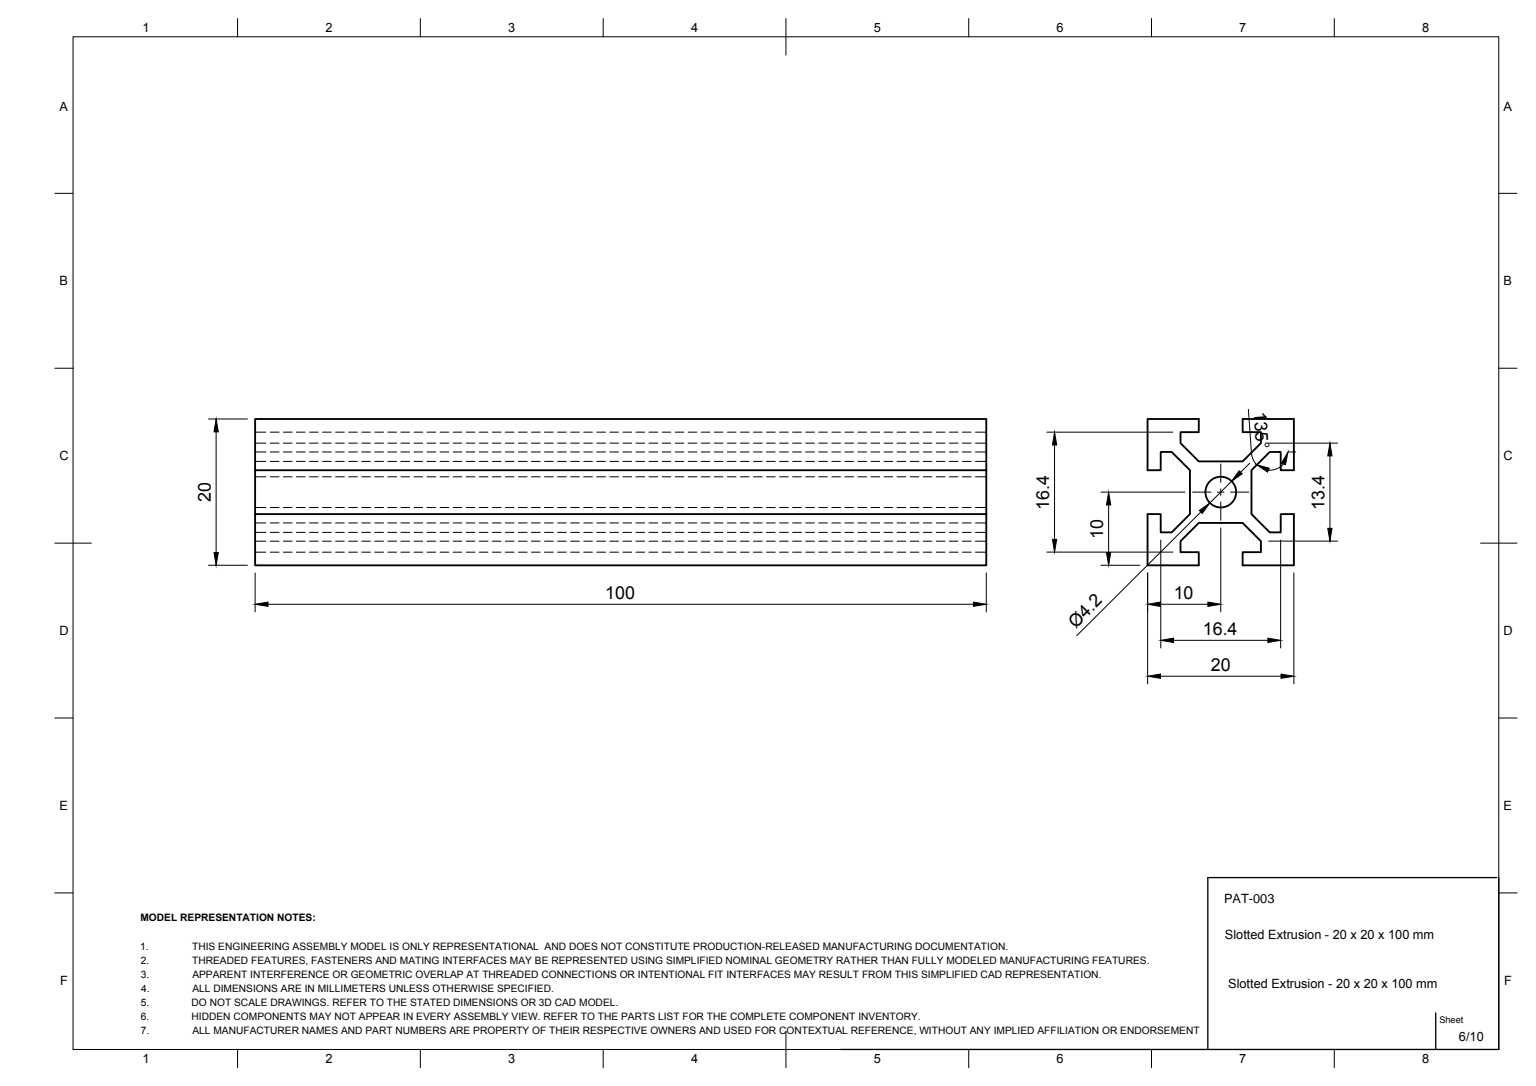
ISO-10303-21;
HEADER;
/* Generated by software containing ST-Developer
 * from STEP Tools, Inc. (www.steptools.com) 
 */

FILE_DESCRIPTION(
/* description */ ('PAT-003'),
/* implementation_level */ '2;1');

FILE_NAME(
/* name */ 'Slotted Extrusion - 20 x 20 x 100 mm.step',
/* time_stamp */ '2026-10-29T15:45:40-07:00',
/* author */ (''),
/* organization */ (''),
/* preprocessor_version */ 'ST-DEVELOPER v20.2',
/* originating_system */ 'Autodesk Translation Framework v15.17.0.0',
/* authorisation */ '');

FILE_SCHEMA (('AUTOMOTIVE_DESIGN { 1 0 10303 214 3 1 1 }'));
ENDSEC;

DATA;
#10=MECHANICAL_DESIGN_GEOMETRIC_PRESENTATION_REPRESENTATION('',(#151),#5761);
#127=SHAPE_REPRESENTATION_RELATIONSHIP('SRR','None',#5821,#139);
#139=ADVANCED_BREP_SHAPE_REPRESENTATION('',(#162),#5752);
#151=STYLED_ITEM('',(#5963),#162);
#162=MANIFOLD_SOLID_BREP('Body1',#3326);
#183=FACE_BOUND('',#640,.T.);
#184=FACE_BOUND('',#642,.T.);
#242=PLANE('',#3559);
#243=PLANE('',#3560);
#244=PLANE('',#3561);
#245=PLANE('',#3562);
#246=PLANE('',#3563);
#247=PLANE('',#3564);
#248=PLANE('',#3565);
#249=PLANE('',#3566);
#250=PLANE('',#3567);
#251=PLANE('',#3568);
#252=PLANE('',#3569);
#253=PLANE('',#3570);
#254=PLANE('',#3571);
#255=PLANE('',#3572);
#256=PLANE('',#3573);
#257=PLANE('',#3574);
#258=PLANE('',#3575);
#259=PLANE('',#3576);
#260=PLANE('',#3577);
#261=PLANE('',#3578);
#262=PLANE('',#3579);
#263=PLANE('',#3580);
#264=PLANE('',#3581);
#265=PLANE('',#3582);
#266=PLANE('',#3583);
#267=PLANE('',#3584);
#268=PLANE('',#3585);
#269=PLANE('',#3586);
#270=PLANE('',#3587);
#271=PLANE('',#3588);
#272=PLANE('',#3589);
#273=PLANE('',#3590);
#274=PLANE('',#3591);
#275=PLANE('',#3592);
#276=PLANE('',#3593);
#277=PLANE('',#3594);
#278=PLANE('',#3598);
#279=PLANE('',#3599);
#280=PLANE('',#3600);
#281=PLANE('',#3601);
#282=PLANE('',#3602);
#283=PLANE('',#3603);
#284=PLANE('',#3604);
#285=PLANE('',#3605);
#286=PLANE('',#3606);
#287=PLANE('',#3607);
#393=FACE_OUTER_BOUND('',#594,.T.);
#394=FACE_OUTER_BOUND('',#595,.T.);
#395=FACE_OUTER_BOUND('',#596,.T.);
#396=FACE_OUTER_BOUND('',#597,.T.);
#397=FACE_OUTER_BOUND('',#598,.T.);
#398=FACE_OUTER_BOUND('',#599,.T.);
#399=FACE_OUTER_BOUND('',#600,.T.);
#400=FACE_OUTER_BOUND('',#601,.T.);
#401=FACE_OUTER_BOUND('',#602,.T.);
#402=FACE_OUTER_BOUND('',#603,.T.);
#403=FACE_OUTER_BOUND('',#604,.T.);
#404=FACE_OUTER_BOUND('',#605,.T.);
#405=FACE_OUTER_BOUND('',#606,.T.);
#406=FACE_OUTER_BOUND('',#607,.T.);
#407=FACE_OUTER_BOUND('',#608,.T.);
#408=FACE_OUTER_BOUND('',#609,.T.);
#409=FACE_OUTER_BOUND('',#610,.T.);
#410=FACE_OUTER_BOUND('',#611,.T.);
#411=FACE_OUTER_BOUND('',#612,.T.);
#412=FACE_OUTER_BOUND('',#613,.T.);
#413=FACE_OUTER_BOUND('',#614,.T.);
#414=FACE_OUTER_BOUND('',#615,.T.);
#415=FACE_OUTER_BOUND('',#616,.T.);
#416=FACE_OUTER_BOUND('',#617,.T.);
#417=FACE_OUTER_BOUND('',#618,.T.);
#418=FACE_OUTER_BOUND('',#619,.T.);
#419=FACE_OUTER_BOUND('',#620,.T.);
#420=FACE_OUTER_BOUND('',#621,.T.);
#421=FACE_OUTER_BOUND('',#622,.T.);
#422=FACE_OUTER_BOUND('',#623,.T.);
#423=FACE_OUTER_BOUND('',#624,.T.);
#424=FACE_OUTER_BOUND('',#625,.T.);
#425=FACE_OUTER_BOUND('',#626,.T.);
#426=FACE_OUTER_BOUND('',#627,.T.);
#427=FACE_OUTER_BOUND('',#628,.T.);
#428=FACE_OUTER_BOUND('',#629,.T.);
#429=FACE_OUTER_BOUND('',#630,.T.);
#430=FACE_OUTER_BOUND('',#631,.T.);
#431=FACE_OUTER_BOUND('',#632,.T.);
#432=FACE_OUTER_BOUND('',#633,.T.);
#433=FACE_OUTER_BOUND('',#634,.T.);
#434=FACE_OUTER_BOUND('',#635,.T.);
#435=FACE_OUTER_BOUND('',#636,.T.);
#436=FACE_OUTER_BOUND('',#637,.T.);
#437=FACE_OUTER_BOUND('',#638,.T.);
#438=FACE_OUTER_BOUND('',#639,.T.);
#439=FACE_OUTER_BOUND('',#641,.T.);
#594=EDGE_LOOP('',(#2438,#2439,#2440,#2441));
#595=EDGE_LOOP('',(#2442,#2443,#2444,#2445));
#596=EDGE_LOOP('',(#2446,#2447,#2448,#2449));
#597=EDGE_LOOP('',(#2450,#2451,#2452,#2453));
#598=EDGE_LOOP('',(#2454,#2455,#2456,#2457));
#599=EDGE_LOOP('',(#2458,#2459,#2460,#2461));
#600=EDGE_LOOP('',(#2462,#2463,#2464,#2465));
#601=EDGE_LOOP('',(#2466,#2467,#2468,#2469));
#602=EDGE_LOOP('',(#2470,#2471,#2472,#2473));
#603=EDGE_LOOP('',(#2474,#2475,#2476,#2477));
#604=EDGE_LOOP('',(#2478,#2479,#2480,#2481));
#605=EDGE_LOOP('',(#2482,#2483,#2484,#2485));
#606=EDGE_LOOP('',(#2486,#2487,#2488,#2489));
#607=EDGE_LOOP('',(#2490,#2491,#2492,#2493));
#608=EDGE_LOOP('',(#2494,#2495,#2496,#2497));
#609=EDGE_LOOP('',(#2498,#2499,#2500,#2501));
#610=EDGE_LOOP('',(#2502,#2503,#2504,#2505));
#611=EDGE_LOOP('',(#2506,#2507,#2508,#2509));
#612=EDGE_LOOP('',(#2510,#2511,#2512,#2513));
#613=EDGE_LOOP('',(#2514,#2515,#2516,#2517));
#614=EDGE_LOOP('',(#2518,#2519,#2520,#2521));
#615=EDGE_LOOP('',(#2522,#2523,#2524,#2525));
#616=EDGE_LOOP('',(#2526,#2527,#2528,#2529));
#617=EDGE_LOOP('',(#2530,#2531,#2532,#2533));
#618=EDGE_LOOP('',(#2534,#2535,#2536,#2537));
#619=EDGE_LOOP('',(#2538,#2539,#2540,#2541));
#620=EDGE_LOOP('',(#2542,#2543,#2544,#2545));
#621=EDGE_LOOP('',(#2546,#2547,#2548,#2549));
#622=EDGE_LOOP('',(#2550,#2551,#2552,#2553));
#623=EDGE_LOOP('',(#2554,#2555,#2556,#2557));
#624=EDGE_LOOP('',(#2558,#2559,#2560,#2561));
#625=EDGE_LOOP('',(#2562,#2563,#2564,#2565));
#626=EDGE_LOOP('',(#2566,#2567,#2568,#2569));
#627=EDGE_LOOP('',(#2570,#2571,#2572,#2573));
#628=EDGE_LOOP('',(#2574,#2575,#2576,#2577));
#629=EDGE_LOOP('',(#2578,#2579,#2580,#2581));
#630=EDGE_LOOP('',(#2582,#2583,#2584,#2585));
#631=EDGE_LOOP('',(#2586,#2587,#2588,#2589));
#632=EDGE_LOOP('',(#2590,#2591,#2592,#2593));
#633=EDGE_LOOP('',(#2594,#2595,#2596,#2597));
#634=EDGE_LOOP('',(#2598,#2599,#2600,#2601));
#635=EDGE_LOOP('',(#2602,#2603,#2604,#2605));
#636=EDGE_LOOP('',(#2606,#2607,#2608,#2609));
#637=EDGE_LOOP('',(#2610,#2611,#2612,#2613));
#638=EDGE_LOOP('',(#2614,#2615,#2616,#2617));
#639=EDGE_LOOP('',(#2618,#2619,#2620,#2621,#2622,#2623,#2624,#2625,#2626,
#2627,#2628,#2629,#2630,#2631,#2632,#2633,#2634,#2635,#2636,#2637,#2638,
#2639,#2640,#2641,#2642,#2643,#2644,#2645,#2646,#2647,#2648,#2649,#2650,
#2651,#2652,#2653,#2654,#2655,#2656,#2657,#2658,#2659,#2660,#2661));
#640=EDGE_LOOP('',(#2662));
#641=EDGE_LOOP('',(#2663,#2664,#2665,#2666,#2667,#2668,#2669,#2670,#2671,
#2672,#2673,#2674,#2675,#2676,#2677,#2678,#2679,#2680,#2681,#2682,#2683,
#2684,#2685,#2686,#2687,#2688,#2689,#2690,#2691,#2692,#2693,#2694,#2695,
#2696,#2697,#2698,#2699,#2700,#2701,#2702,#2703,#2704,#2705,#2706));
#642=EDGE_LOOP('',(#2707));
#830=LINE('',#4991,#1152);
#831=LINE('',#4993,#1153);
#832=LINE('',#4995,#1154);
#833=LINE('',#4996,#1155);
#834=LINE('',#4999,#1156);
#835=LINE('',#5001,#1157);
#836=LINE('',#5002,#1158);
#837=LINE('',#5005,#1159);
#838=LINE('',#5007,#1160);
#839=LINE('',#5008,#1161);
#840=LINE('',#5011,#1162);
#841=LINE('',#5013,#1163);
#842=LINE('',#5014,#1164);
#843=LINE('',#5017,#1165);
#844=LINE('',#5019,#1166);
#845=LINE('',#5020,#1167);
#846=LINE('',#5023,#1168);
#847=LINE('',#5025,#1169);
#848=LINE('',#5026,#1170);
#849=LINE('',#5029,#1171);
#850=LINE('',#5031,#1172);
#851=LINE('',#5032,#1173);
#852=LINE('',#5035,#1174);
#853=LINE('',#5037,#1175);
#854=LINE('',#5038,#1176);
#855=LINE('',#5041,#1177);
#856=LINE('',#5043,#1178);
#857=LINE('',#5044,#1179);
#858=LINE('',#5048,#1180);
#859=LINE('',#5050,#1181);
#860=LINE('',#5052,#1182);
#861=LINE('',#5053,#1183);
#862=LINE('',#5056,#1184);
#863=LINE('',#5058,#1185);
#864=LINE('',#5059,#1186);
#865=LINE('',#5062,#1187);
#866=LINE('',#5064,#1188);
#867=LINE('',#5065,#1189);
#868=LINE('',#5068,#1190);
#869=LINE('',#5070,#1191);
#870=LINE('',#5071,#1192);
#871=LINE('',#5074,#1193);
#872=LINE('',#5076,#1194);
#873=LINE('',#5077,#1195);
#874=LINE('',#5080,#1196);
#875=LINE('',#5082,#1197);
#876=LINE('',#5083,#1198);
#877=LINE('',#5086,#1199);
#878=LINE('',#5088,#1200);
#879=LINE('',#5089,#1201);
#880=LINE('',#5092,#1202);
#881=LINE('',#5094,#1203);
#882=LINE('',#5095,#1204);
#883=LINE('',#5098,#1205);
#884=LINE('',#5100,#1206);
#885=LINE('',#5101,#1207);
#886=LINE('',#5105,#1208);
#887=LINE('',#5107,#1209);
#888=LINE('',#5109,#1210);
#889=LINE('',#5110,#1211);
#890=LINE('',#5113,#1212);
#891=LINE('',#5115,#1213);
#892=LINE('',#5116,#1214);
#893=LINE('',#5119,#1215);
#894=LINE('',#5121,#1216);
#895=LINE('',#5122,#1217);
#896=LINE('',#5125,#1218);
#897=LINE('',#5127,#1219);
#898=LINE('',#5128,#1220);
#899=LINE('',#5131,#1221);
#900=LINE('',#5133,#1222);
#901=LINE('',#5134,#1223);
#902=LINE('',#5137,#1224);
#903=LINE('',#5139,#1225);
#904=LINE('',#5140,#1226);
#905=LINE('',#5143,#1227);
#906=LINE('',#5145,#1228);
#907=LINE('',#5146,#1229);
#908=LINE('',#5149,#1230);
#909=LINE('',#5151,#1231);
#910=LINE('',#5152,#1232);
#911=LINE('',#5155,#1233);
#912=LINE('',#5157,#1234);
#913=LINE('',#5158,#1235);
#914=LINE('',#5162,#1236);
#915=LINE('',#5164,#1237);
#916=LINE('',#5166,#1238);
#917=LINE('',#5167,#1239);
#918=LINE('',#5170,#1240);
#919=LINE('',#5172,#1241);
#920=LINE('',#5173,#1242);
#921=LINE('',#5176,#1243);
#922=LINE('',#5178,#1244);
#923=LINE('',#5179,#1245);
#924=LINE('',#5182,#1246);
#925=LINE('',#5184,#1247);
#926=LINE('',#5185,#1248);
#927=LINE('',#5188,#1249);
#928=LINE('',#5190,#1250);
#929=LINE('',#5191,#1251);
#930=LINE('',#5194,#1252);
#931=LINE('',#5196,#1253);
#932=LINE('',#5197,#1254);
#933=LINE('',#5200,#1255);
#934=LINE('',#5202,#1256);
#935=LINE('',#5203,#1257);
#936=LINE('',#5206,#1258);
#937=LINE('',#5208,#1259);
#938=LINE('',#5209,#1260);
#939=LINE('',#5212,#1261);
#940=LINE('',#5214,#1262);
#941=LINE('',#5215,#1263);
#942=LINE('',#5220,#1264);
#943=LINE('',#5224,#1265);
#944=LINE('',#5226,#1266);
#945=LINE('',#5227,#1267);
#946=LINE('',#5230,#1268);
#947=LINE('',#5232,#1269);
#948=LINE('',#5233,#1270);
#949=LINE('',#5235,#1271);
#950=LINE('',#5236,#1272);
#951=LINE('',#5239,#1273);
#952=LINE('',#5241,#1274);
#953=LINE('',#5242,#1275);
#954=LINE('',#5244,#1276);
#955=LINE('',#5245,#1277);
#956=LINE('',#5248,#1278);
#957=LINE('',#5250,#1279);
#958=LINE('',#5251,#1280);
#959=LINE('',#5253,#1281);
#960=LINE('',#5254,#1282);
#961=LINE('',#5256,#1283);
#962=LINE('',#5257,#1284);
#1152=VECTOR('',#4049,1.);
#1153=VECTOR('',#4050,1.);
#1154=VECTOR('',#4051,1.);
#1155=VECTOR('',#4052,1.);
#1156=VECTOR('',#4055,1.);
#1157=VECTOR('',#4056,1.);
#1158=VECTOR('',#4057,1.);
#1159=VECTOR('',#4060,1.);
#1160=VECTOR('',#4061,1.);
#1161=VECTOR('',#4062,1.);
#1162=VECTOR('',#4065,1.);
#1163=VECTOR('',#4066,1.);
#1164=VECTOR('',#4067,1.);
#1165=VECTOR('',#4070,1.);
#1166=VECTOR('',#4071,1.);
#1167=VECTOR('',#4072,1.);
#1168=VECTOR('',#4075,1.);
#1169=VECTOR('',#4076,1.);
#1170=VECTOR('',#4077,1.);
#1171=VECTOR('',#4080,1.);
#1172=VECTOR('',#4081,1.);
#1173=VECTOR('',#4082,1.);
#1174=VECTOR('',#4085,1.);
#1175=VECTOR('',#4086,1.);
#1176=VECTOR('',#4087,1.);
#1177=VECTOR('',#4090,1.);
#1178=VECTOR('',#4091,1.);
#1179=VECTOR('',#4092,1.);
#1180=VECTOR('',#4095,1.);
#1181=VECTOR('',#4096,1.);
#1182=VECTOR('',#4097,1.);
#1183=VECTOR('',#4098,1.);
#1184=VECTOR('',#4101,1.);
#1185=VECTOR('',#4102,1.);
#1186=VECTOR('',#4103,1.);
#1187=VECTOR('',#4106,1.);
#1188=VECTOR('',#4107,1.);
#1189=VECTOR('',#4108,1.);
#1190=VECTOR('',#4111,1.);
#1191=VECTOR('',#4112,1.);
#1192=VECTOR('',#4113,1.);
#1193=VECTOR('',#4116,1.);
#1194=VECTOR('',#4117,1.);
#1195=VECTOR('',#4118,1.);
#1196=VECTOR('',#4121,1.);
#1197=VECTOR('',#4122,1.);
#1198=VECTOR('',#4123,1.);
#1199=VECTOR('',#4126,1.);
#1200=VECTOR('',#4127,1.);
#1201=VECTOR('',#4128,1.);
#1202=VECTOR('',#4131,1.);
#1203=VECTOR('',#4132,1.);
#1204=VECTOR('',#4133,1.);
#1205=VECTOR('',#4136,1.);
#1206=VECTOR('',#4137,1.);
#1207=VECTOR('',#4138,1.);
#1208=VECTOR('',#4141,1.);
#1209=VECTOR('',#4142,1.);
#1210=VECTOR('',#4143,1.);
#1211=VECTOR('',#4144,1.);
#1212=VECTOR('',#4147,1.);
#1213=VECTOR('',#4148,1.);
#1214=VECTOR('',#4149,1.);
#1215=VECTOR('',#4152,1.);
#1216=VECTOR('',#4153,1.);
#1217=VECTOR('',#4154,1.);
#1218=VECTOR('',#4157,1.);
#1219=VECTOR('',#4158,1.);
#1220=VECTOR('',#4159,1.);
#1221=VECTOR('',#4162,1.);
#1222=VECTOR('',#4163,1.);
#1223=VECTOR('',#4164,1.);
#1224=VECTOR('',#4167,1.);
#1225=VECTOR('',#4168,1.);
#1226=VECTOR('',#4169,1.);
#1227=VECTOR('',#4172,1.);
#1228=VECTOR('',#4173,1.);
#1229=VECTOR('',#4174,1.);
#1230=VECTOR('',#4177,1.);
#1231=VECTOR('',#4178,1.);
#1232=VECTOR('',#4179,1.);
#1233=VECTOR('',#4182,1.);
#1234=VECTOR('',#4183,1.);
#1235=VECTOR('',#4184,1.);
#1236=VECTOR('',#4187,1.);
#1237=VECTOR('',#4188,1.);
#1238=VECTOR('',#4189,1.);
#1239=VECTOR('',#4190,1.);
#1240=VECTOR('',#4193,1.);
#1241=VECTOR('',#4194,1.);
#1242=VECTOR('',#4195,1.);
#1243=VECTOR('',#4198,1.);
#1244=VECTOR('',#4199,1.);
#1245=VECTOR('',#4200,1.);
#1246=VECTOR('',#4203,1.);
#1247=VECTOR('',#4204,1.);
#1248=VECTOR('',#4205,1.);
#1249=VECTOR('',#4208,1.);
#1250=VECTOR('',#4209,1.);
#1251=VECTOR('',#4210,1.);
#1252=VECTOR('',#4213,1.);
#1253=VECTOR('',#4214,1.);
#1254=VECTOR('',#4215,1.);
#1255=VECTOR('',#4218,1.);
#1256=VECTOR('',#4219,1.);
#1257=VECTOR('',#4220,1.);
#1258=VECTOR('',#4223,1.);
#1259=VECTOR('',#4224,1.);
#1260=VECTOR('',#4225,1.);
#1261=VECTOR('',#4228,1.);
#1262=VECTOR('',#4229,1.);
#1263=VECTOR('',#4230,1.);
#1264=VECTOR('',#4235,0.21);
#1265=VECTOR('',#4240,1.);
#1266=VECTOR('',#4241,1.);
#1267=VECTOR('',#4242,1.);
#1268=VECTOR('',#4245,1.);
#1269=VECTOR('',#4246,1.);
#1270=VECTOR('',#4247,1.);
#1271=VECTOR('',#4250,1.);
#1272=VECTOR('',#4251,1.);
#1273=VECTOR('',#4254,1.);
#1274=VECTOR('',#4255,1.);
#1275=VECTOR('',#4256,1.);
#1276=VECTOR('',#4259,1.);
#1277=VECTOR('',#4260,1.);
#1278=VECTOR('',#4263,1.);
#1279=VECTOR('',#4264,1.);
#1280=VECTOR('',#4265,1.);
#1281=VECTOR('',#4268,1.);
#1282=VECTOR('',#4269,1.);
#1283=VECTOR('',#4272,1.);
#1284=VECTOR('',#4273,1.);
#1426=CIRCLE('',#3596,0.21);
#1427=CIRCLE('',#3597,0.21);
#1564=VERTEX_POINT('',#4989);
#1565=VERTEX_POINT('',#4990);
#1566=VERTEX_POINT('',#4992);
#1567=VERTEX_POINT('',#4994);
#1568=VERTEX_POINT('',#4998);
#1569=VERTEX_POINT('',#5000);
#1570=VERTEX_POINT('',#5004);
#1571=VERTEX_POINT('',#5006);
#1572=VERTEX_POINT('',#5010);
#1573=VERTEX_POINT('',#5012);
#1574=VERTEX_POINT('',#5016);
#1575=VERTEX_POINT('',#5018);
#1576=VERTEX_POINT('',#5022);
#1577=VERTEX_POINT('',#5024);
#1578=VERTEX_POINT('',#5028);
#1579=VERTEX_POINT('',#5030);
#1580=VERTEX_POINT('',#5034);
#1581=VERTEX_POINT('',#5036);
#1582=VERTEX_POINT('',#5040);
#1583=VERTEX_POINT('',#5042);
#1584=VERTEX_POINT('',#5046);
#1585=VERTEX_POINT('',#5047);
#1586=VERTEX_POINT('',#5049);
#1587=VERTEX_POINT('',#5051);
#1588=VERTEX_POINT('',#5055);
#1589=VERTEX_POINT('',#5057);
#1590=VERTEX_POINT('',#5061);
#1591=VERTEX_POINT('',#5063);
#1592=VERTEX_POINT('',#5067);
#1593=VERTEX_POINT('',#5069);
#1594=VERTEX_POINT('',#5073);
#1595=VERTEX_POINT('',#5075);
#1596=VERTEX_POINT('',#5079);
#1597=VERTEX_POINT('',#5081);
#1598=VERTEX_POINT('',#5085);
#1599=VERTEX_POINT('',#5087);
#1600=VERTEX_POINT('',#5091);
#1601=VERTEX_POINT('',#5093);
#1602=VERTEX_POINT('',#5097);
#1603=VERTEX_POINT('',#5099);
#1604=VERTEX_POINT('',#5103);
#1605=VERTEX_POINT('',#5104);
#1606=VERTEX_POINT('',#5106);
#1607=VERTEX_POINT('',#5108);
#1608=VERTEX_POINT('',#5112);
#1609=VERTEX_POINT('',#5114);
#1610=VERTEX_POINT('',#5118);
#1611=VERTEX_POINT('',#5120);
#1612=VERTEX_POINT('',#5124);
#1613=VERTEX_POINT('',#5126);
#1614=VERTEX_POINT('',#5130);
#1615=VERTEX_POINT('',#5132);
#1616=VERTEX_POINT('',#5136);
#1617=VERTEX_POINT('',#5138);
#1618=VERTEX_POINT('',#5142);
#1619=VERTEX_POINT('',#5144);
#1620=VERTEX_POINT('',#5148);
#1621=VERTEX_POINT('',#5150);
#1622=VERTEX_POINT('',#5154);
#1623=VERTEX_POINT('',#5156);
#1624=VERTEX_POINT('',#5160);
#1625=VERTEX_POINT('',#5161);
#1626=VERTEX_POINT('',#5163);
#1627=VERTEX_POINT('',#5165);
#1628=VERTEX_POINT('',#5169);
#1629=VERTEX_POINT('',#5171);
#1630=VERTEX_POINT('',#5175);
#1631=VERTEX_POINT('',#5177);
#1632=VERTEX_POINT('',#5181);
#1633=VERTEX_POINT('',#5183);
#1634=VERTEX_POINT('',#5187);
#1635=VERTEX_POINT('',#5189);
#1636=VERTEX_POINT('',#5193);
#1637=VERTEX_POINT('',#5195);
#1638=VERTEX_POINT('',#5199);
#1639=VERTEX_POINT('',#5201);
#1640=VERTEX_POINT('',#5205);
#1641=VERTEX_POINT('',#5207);
#1642=VERTEX_POINT('',#5211);
#1643=VERTEX_POINT('',#5213);
#1644=VERTEX_POINT('',#5217);
#1645=VERTEX_POINT('',#5219);
#1646=VERTEX_POINT('',#5223);
#1647=VERTEX_POINT('',#5225);
#1648=VERTEX_POINT('',#5229);
#1649=VERTEX_POINT('',#5231);
#1650=VERTEX_POINT('',#5238);
#1651=VERTEX_POINT('',#5240);
#1652=VERTEX_POINT('',#5247);
#1653=VERTEX_POINT('',#5249);
#1890=EDGE_CURVE('',#1564,#1565,#830,.T.);
#1891=EDGE_CURVE('',#1564,#1566,#831,.T.);
#1892=EDGE_CURVE('',#1567,#1566,#832,.T.);
#1893=EDGE_CURVE('',#1565,#1567,#833,.T.);
#1894=EDGE_CURVE('',#1568,#1564,#834,.T.);
#1895=EDGE_CURVE('',#1568,#1569,#835,.T.);
#1896=EDGE_CURVE('',#1566,#1569,#836,.T.);
#1897=EDGE_CURVE('',#1570,#1568,#837,.T.);
#1898=EDGE_CURVE('',#1570,#1571,#838,.T.);
#1899=EDGE_CURVE('',#1569,#1571,#839,.T.);
#1900=EDGE_CURVE('',#1572,#1570,#840,.T.);
#1901=EDGE_CURVE('',#1572,#1573,#841,.T.);
#1902=EDGE_CURVE('',#1571,#1573,#842,.T.);
#1903=EDGE_CURVE('',#1574,#1572,#843,.T.);
#1904=EDGE_CURVE('',#1574,#1575,#844,.T.);
#1905=EDGE_CURVE('',#1573,#1575,#845,.T.);
#1906=EDGE_CURVE('',#1576,#1574,#846,.T.);
#1907=EDGE_CURVE('',#1576,#1577,#847,.T.);
#1908=EDGE_CURVE('',#1575,#1577,#848,.T.);
#1909=EDGE_CURVE('',#1578,#1576,#849,.T.);
#1910=EDGE_CURVE('',#1578,#1579,#850,.T.);
#1911=EDGE_CURVE('',#1577,#1579,#851,.T.);
#1912=EDGE_CURVE('',#1580,#1578,#852,.T.);
#1913=EDGE_CURVE('',#1580,#1581,#853,.T.);
#1914=EDGE_CURVE('',#1579,#1581,#854,.T.);
#1915=EDGE_CURVE('',#1582,#1580,#855,.T.);
#1916=EDGE_CURVE('',#1583,#1582,#856,.T.);
#1917=EDGE_CURVE('',#1581,#1583,#857,.T.);
#1918=EDGE_CURVE('',#1584,#1585,#858,.T.);
#1919=EDGE_CURVE('',#1584,#1586,#859,.T.);
#1920=EDGE_CURVE('',#1587,#1586,#860,.T.);
#1921=EDGE_CURVE('',#1585,#1587,#861,.T.);
#1922=EDGE_CURVE('',#1588,#1584,#862,.T.);
#1923=EDGE_CURVE('',#1588,#1589,#863,.T.);
#1924=EDGE_CURVE('',#1586,#1589,#864,.T.);
#1925=EDGE_CURVE('',#1590,#1588,#865,.T.);
#1926=EDGE_CURVE('',#1590,#1591,#866,.T.);
#1927=EDGE_CURVE('',#1589,#1591,#867,.T.);
#1928=EDGE_CURVE('',#1592,#1590,#868,.T.);
#1929=EDGE_CURVE('',#1592,#1593,#869,.T.);
#1930=EDGE_CURVE('',#1591,#1593,#870,.T.);
#1931=EDGE_CURVE('',#1594,#1592,#871,.T.);
#1932=EDGE_CURVE('',#1594,#1595,#872,.T.);
#1933=EDGE_CURVE('',#1593,#1595,#873,.T.);
#1934=EDGE_CURVE('',#1596,#1594,#874,.T.);
#1935=EDGE_CURVE('',#1596,#1597,#875,.T.);
#1936=EDGE_CURVE('',#1595,#1597,#876,.T.);
#1937=EDGE_CURVE('',#1598,#1596,#877,.T.);
#1938=EDGE_CURVE('',#1598,#1599,#878,.T.);
#1939=EDGE_CURVE('',#1597,#1599,#879,.T.);
#1940=EDGE_CURVE('',#1600,#1598,#880,.T.);
#1941=EDGE_CURVE('',#1600,#1601,#881,.T.);
#1942=EDGE_CURVE('',#1599,#1601,#882,.T.);
#1943=EDGE_CURVE('',#1602,#1600,#883,.T.);
#1944=EDGE_CURVE('',#1603,#1602,#884,.T.);
#1945=EDGE_CURVE('',#1601,#1603,#885,.T.);
#1946=EDGE_CURVE('',#1604,#1605,#886,.T.);
#1947=EDGE_CURVE('',#1604,#1606,#887,.T.);
#1948=EDGE_CURVE('',#1607,#1606,#888,.T.);
#1949=EDGE_CURVE('',#1605,#1607,#889,.T.);
#1950=EDGE_CURVE('',#1608,#1604,#890,.T.);
#1951=EDGE_CURVE('',#1608,#1609,#891,.T.);
#1952=EDGE_CURVE('',#1606,#1609,#892,.T.);
#1953=EDGE_CURVE('',#1610,#1608,#893,.T.);
#1954=EDGE_CURVE('',#1610,#1611,#894,.T.);
#1955=EDGE_CURVE('',#1609,#1611,#895,.T.);
#1956=EDGE_CURVE('',#1612,#1610,#896,.T.);
#1957=EDGE_CURVE('',#1612,#1613,#897,.T.);
#1958=EDGE_CURVE('',#1611,#1613,#898,.T.);
#1959=EDGE_CURVE('',#1614,#1612,#899,.T.);
#1960=EDGE_CURVE('',#1614,#1615,#900,.T.);
#1961=EDGE_CURVE('',#1613,#1615,#901,.T.);
#1962=EDGE_CURVE('',#1616,#1614,#902,.T.);
#1963=EDGE_CURVE('',#1616,#1617,#903,.T.);
#1964=EDGE_CURVE('',#1615,#1617,#904,.T.);
#1965=EDGE_CURVE('',#1618,#1616,#905,.T.);
#1966=EDGE_CURVE('',#1618,#1619,#906,.T.);
#1967=EDGE_CURVE('',#1617,#1619,#907,.T.);
#1968=EDGE_CURVE('',#1620,#1618,#908,.T.);
#1969=EDGE_CURVE('',#1620,#1621,#909,.T.);
#1970=EDGE_CURVE('',#1619,#1621,#910,.T.);
#1971=EDGE_CURVE('',#1622,#1620,#911,.T.);
#1972=EDGE_CURVE('',#1623,#1622,#912,.T.);
#1973=EDGE_CURVE('',#1621,#1623,#913,.T.);
#1974=EDGE_CURVE('',#1624,#1625,#914,.T.);
#1975=EDGE_CURVE('',#1624,#1626,#915,.T.);
#1976=EDGE_CURVE('',#1627,#1626,#916,.T.);
#1977=EDGE_CURVE('',#1625,#1627,#917,.T.);
#1978=EDGE_CURVE('',#1628,#1624,#918,.T.);
#1979=EDGE_CURVE('',#1628,#1629,#919,.T.);
#1980=EDGE_CURVE('',#1626,#1629,#920,.T.);
#1981=EDGE_CURVE('',#1630,#1628,#921,.T.);
#1982=EDGE_CURVE('',#1630,#1631,#922,.T.);
#1983=EDGE_CURVE('',#1629,#1631,#923,.T.);
#1984=EDGE_CURVE('',#1632,#1630,#924,.T.);
#1985=EDGE_CURVE('',#1632,#1633,#925,.T.);
#1986=EDGE_CURVE('',#1631,#1633,#926,.T.);
#1987=EDGE_CURVE('',#1634,#1632,#927,.T.);
#1988=EDGE_CURVE('',#1634,#1635,#928,.T.);
#1989=EDGE_CURVE('',#1633,#1635,#929,.T.);
#1990=EDGE_CURVE('',#1636,#1634,#930,.T.);
#1991=EDGE_CURVE('',#1636,#1637,#931,.T.);
#1992=EDGE_CURVE('',#1635,#1637,#932,.T.);
#1993=EDGE_CURVE('',#1638,#1636,#933,.T.);
#1994=EDGE_CURVE('',#1638,#1639,#934,.T.);
#1995=EDGE_CURVE('',#1637,#1639,#935,.T.);
#1996=EDGE_CURVE('',#1640,#1638,#936,.T.);
#1997=EDGE_CURVE('',#1640,#1641,#937,.T.);
#1998=EDGE_CURVE('',#1639,#1641,#938,.T.);
#1999=EDGE_CURVE('',#1642,#1640,#939,.T.);
#2000=EDGE_CURVE('',#1643,#1642,#940,.T.);
#2001=EDGE_CURVE('',#1641,#1643,#941,.T.);
#2002=EDGE_CURVE('',#1644,#1644,#1426,.T.);
#2003=EDGE_CURVE('',#1644,#1645,#942,.T.);
#2004=EDGE_CURVE('',#1645,#1645,#1427,.T.);
#2005=EDGE_CURVE('',#1582,#1646,#943,.T.);
#2006=EDGE_CURVE('',#1646,#1647,#944,.T.);
#2007=EDGE_CURVE('',#1583,#1647,#945,.T.);
#2008=EDGE_CURVE('',#1648,#1567,#946,.T.);
#2009=EDGE_CURVE('',#1649,#1648,#947,.T.);
#2010=EDGE_CURVE('',#1649,#1565,#948,.T.);
#2011=EDGE_CURVE('',#1602,#1649,#949,.T.);
#2012=EDGE_CURVE('',#1603,#1648,#950,.T.);
#2013=EDGE_CURVE('',#1650,#1587,#951,.T.);
#2014=EDGE_CURVE('',#1651,#1650,#952,.T.);
#2015=EDGE_CURVE('',#1651,#1585,#953,.T.);
#2016=EDGE_CURVE('',#1622,#1651,#954,.T.);
#2017=EDGE_CURVE('',#1623,#1650,#955,.T.);
#2018=EDGE_CURVE('',#1652,#1607,#956,.T.);
#2019=EDGE_CURVE('',#1653,#1652,#957,.T.);
#2020=EDGE_CURVE('',#1653,#1605,#958,.T.);
#2021=EDGE_CURVE('',#1642,#1653,#959,.T.);
#2022=EDGE_CURVE('',#1643,#1652,#960,.T.);
#2023=EDGE_CURVE('',#1647,#1627,#961,.T.);
#2024=EDGE_CURVE('',#1646,#1625,#962,.T.);
#2438=ORIENTED_EDGE('',*,*,#1890,.F.);
#2439=ORIENTED_EDGE('',*,*,#1891,.T.);
#2440=ORIENTED_EDGE('',*,*,#1892,.F.);
#2441=ORIENTED_EDGE('',*,*,#1893,.F.);
#2442=ORIENTED_EDGE('',*,*,#1894,.F.);
#2443=ORIENTED_EDGE('',*,*,#1895,.T.);
#2444=ORIENTED_EDGE('',*,*,#1896,.F.);
#2445=ORIENTED_EDGE('',*,*,#1891,.F.);
#2446=ORIENTED_EDGE('',*,*,#1897,.F.);
#2447=ORIENTED_EDGE('',*,*,#1898,.T.);
#2448=ORIENTED_EDGE('',*,*,#1899,.F.);
#2449=ORIENTED_EDGE('',*,*,#1895,.F.);
#2450=ORIENTED_EDGE('',*,*,#1900,.F.);
#2451=ORIENTED_EDGE('',*,*,#1901,.T.);
#2452=ORIENTED_EDGE('',*,*,#1902,.F.);
#2453=ORIENTED_EDGE('',*,*,#1898,.F.);
#2454=ORIENTED_EDGE('',*,*,#1903,.F.);
#2455=ORIENTED_EDGE('',*,*,#1904,.T.);
#2456=ORIENTED_EDGE('',*,*,#1905,.F.);
#2457=ORIENTED_EDGE('',*,*,#1901,.F.);
#2458=ORIENTED_EDGE('',*,*,#1906,.F.);
#2459=ORIENTED_EDGE('',*,*,#1907,.T.);
#2460=ORIENTED_EDGE('',*,*,#1908,.F.);
#2461=ORIENTED_EDGE('',*,*,#1904,.F.);
#2462=ORIENTED_EDGE('',*,*,#1909,.F.);
#2463=ORIENTED_EDGE('',*,*,#1910,.T.);
#2464=ORIENTED_EDGE('',*,*,#1911,.F.);
#2465=ORIENTED_EDGE('',*,*,#1907,.F.);
#2466=ORIENTED_EDGE('',*,*,#1912,.F.);
#2467=ORIENTED_EDGE('',*,*,#1913,.T.);
#2468=ORIENTED_EDGE('',*,*,#1914,.F.);
#2469=ORIENTED_EDGE('',*,*,#1910,.F.);
#2470=ORIENTED_EDGE('',*,*,#1915,.F.);
#2471=ORIENTED_EDGE('',*,*,#1916,.F.);
#2472=ORIENTED_EDGE('',*,*,#1917,.F.);
#2473=ORIENTED_EDGE('',*,*,#1913,.F.);
#2474=ORIENTED_EDGE('',*,*,#1918,.F.);
#2475=ORIENTED_EDGE('',*,*,#1919,.T.);
#2476=ORIENTED_EDGE('',*,*,#1920,.F.);
#2477=ORIENTED_EDGE('',*,*,#1921,.F.);
#2478=ORIENTED_EDGE('',*,*,#1922,.F.);
#2479=ORIENTED_EDGE('',*,*,#1923,.T.);
#2480=ORIENTED_EDGE('',*,*,#1924,.F.);
#2481=ORIENTED_EDGE('',*,*,#1919,.F.);
#2482=ORIENTED_EDGE('',*,*,#1925,.F.);
#2483=ORIENTED_EDGE('',*,*,#1926,.T.);
#2484=ORIENTED_EDGE('',*,*,#1927,.F.);
#2485=ORIENTED_EDGE('',*,*,#1923,.F.);
#2486=ORIENTED_EDGE('',*,*,#1928,.F.);
#2487=ORIENTED_EDGE('',*,*,#1929,.T.);
#2488=ORIENTED_EDGE('',*,*,#1930,.F.);
#2489=ORIENTED_EDGE('',*,*,#1926,.F.);
#2490=ORIENTED_EDGE('',*,*,#1931,.F.);
#2491=ORIENTED_EDGE('',*,*,#1932,.T.);
#2492=ORIENTED_EDGE('',*,*,#1933,.F.);
#2493=ORIENTED_EDGE('',*,*,#1929,.F.);
#2494=ORIENTED_EDGE('',*,*,#1934,.F.);
#2495=ORIENTED_EDGE('',*,*,#1935,.T.);
#2496=ORIENTED_EDGE('',*,*,#1936,.F.);
#2497=ORIENTED_EDGE('',*,*,#1932,.F.);
#2498=ORIENTED_EDGE('',*,*,#1937,.F.);
#2499=ORIENTED_EDGE('',*,*,#1938,.T.);
#2500=ORIENTED_EDGE('',*,*,#1939,.F.);
#2501=ORIENTED_EDGE('',*,*,#1935,.F.);
#2502=ORIENTED_EDGE('',*,*,#1940,.F.);
#2503=ORIENTED_EDGE('',*,*,#1941,.T.);
#2504=ORIENTED_EDGE('',*,*,#1942,.F.);
#2505=ORIENTED_EDGE('',*,*,#1938,.F.);
#2506=ORIENTED_EDGE('',*,*,#1943,.F.);
#2507=ORIENTED_EDGE('',*,*,#1944,.F.);
#2508=ORIENTED_EDGE('',*,*,#1945,.F.);
#2509=ORIENTED_EDGE('',*,*,#1941,.F.);
#2510=ORIENTED_EDGE('',*,*,#1946,.F.);
#2511=ORIENTED_EDGE('',*,*,#1947,.T.);
#2512=ORIENTED_EDGE('',*,*,#1948,.F.);
#2513=ORIENTED_EDGE('',*,*,#1949,.F.);
#2514=ORIENTED_EDGE('',*,*,#1950,.F.);
#2515=ORIENTED_EDGE('',*,*,#1951,.T.);
#2516=ORIENTED_EDGE('',*,*,#1952,.F.);
#2517=ORIENTED_EDGE('',*,*,#1947,.F.);
#2518=ORIENTED_EDGE('',*,*,#1953,.F.);
#2519=ORIENTED_EDGE('',*,*,#1954,.T.);
#2520=ORIENTED_EDGE('',*,*,#1955,.F.);
#2521=ORIENTED_EDGE('',*,*,#1951,.F.);
#2522=ORIENTED_EDGE('',*,*,#1956,.F.);
#2523=ORIENTED_EDGE('',*,*,#1957,.T.);
#2524=ORIENTED_EDGE('',*,*,#1958,.F.);
#2525=ORIENTED_EDGE('',*,*,#1954,.F.);
#2526=ORIENTED_EDGE('',*,*,#1959,.F.);
#2527=ORIENTED_EDGE('',*,*,#1960,.T.);
#2528=ORIENTED_EDGE('',*,*,#1961,.F.);
#2529=ORIENTED_EDGE('',*,*,#1957,.F.);
#2530=ORIENTED_EDGE('',*,*,#1962,.F.);
#2531=ORIENTED_EDGE('',*,*,#1963,.T.);
#2532=ORIENTED_EDGE('',*,*,#1964,.F.);
#2533=ORIENTED_EDGE('',*,*,#1960,.F.);
#2534=ORIENTED_EDGE('',*,*,#1965,.F.);
#2535=ORIENTED_EDGE('',*,*,#1966,.T.);
#2536=ORIENTED_EDGE('',*,*,#1967,.F.);
#2537=ORIENTED_EDGE('',*,*,#1963,.F.);
#2538=ORIENTED_EDGE('',*,*,#1968,.F.);
#2539=ORIENTED_EDGE('',*,*,#1969,.T.);
#2540=ORIENTED_EDGE('',*,*,#1970,.F.);
#2541=ORIENTED_EDGE('',*,*,#1966,.F.);
#2542=ORIENTED_EDGE('',*,*,#1971,.F.);
#2543=ORIENTED_EDGE('',*,*,#1972,.F.);
#2544=ORIENTED_EDGE('',*,*,#1973,.F.);
#2545=ORIENTED_EDGE('',*,*,#1969,.F.);
#2546=ORIENTED_EDGE('',*,*,#1974,.F.);
#2547=ORIENTED_EDGE('',*,*,#1975,.T.);
#2548=ORIENTED_EDGE('',*,*,#1976,.F.);
#2549=ORIENTED_EDGE('',*,*,#1977,.F.);
#2550=ORIENTED_EDGE('',*,*,#1978,.F.);
#2551=ORIENTED_EDGE('',*,*,#1979,.T.);
#2552=ORIENTED_EDGE('',*,*,#1980,.F.);
#2553=ORIENTED_EDGE('',*,*,#1975,.F.);
#2554=ORIENTED_EDGE('',*,*,#1981,.F.);
#2555=ORIENTED_EDGE('',*,*,#1982,.T.);
#2556=ORIENTED_EDGE('',*,*,#1983,.F.);
#2557=ORIENTED_EDGE('',*,*,#1979,.F.);
#2558=ORIENTED_EDGE('',*,*,#1984,.F.);
#2559=ORIENTED_EDGE('',*,*,#1985,.T.);
#2560=ORIENTED_EDGE('',*,*,#1986,.F.);
#2561=ORIENTED_EDGE('',*,*,#1982,.F.);
#2562=ORIENTED_EDGE('',*,*,#1987,.F.);
#2563=ORIENTED_EDGE('',*,*,#1988,.T.);
#2564=ORIENTED_EDGE('',*,*,#1989,.F.);
#2565=ORIENTED_EDGE('',*,*,#1985,.F.);
#2566=ORIENTED_EDGE('',*,*,#1990,.F.);
#2567=ORIENTED_EDGE('',*,*,#1991,.T.);
#2568=ORIENTED_EDGE('',*,*,#1992,.F.);
#2569=ORIENTED_EDGE('',*,*,#1988,.F.);
#2570=ORIENTED_EDGE('',*,*,#1993,.F.);
#2571=ORIENTED_EDGE('',*,*,#1994,.T.);
#2572=ORIENTED_EDGE('',*,*,#1995,.F.);
#2573=ORIENTED_EDGE('',*,*,#1991,.F.);
#2574=ORIENTED_EDGE('',*,*,#1996,.F.);
#2575=ORIENTED_EDGE('',*,*,#1997,.T.);
#2576=ORIENTED_EDGE('',*,*,#1998,.F.);
#2577=ORIENTED_EDGE('',*,*,#1994,.F.);
#2578=ORIENTED_EDGE('',*,*,#1999,.F.);
#2579=ORIENTED_EDGE('',*,*,#2000,.F.);
#2580=ORIENTED_EDGE('',*,*,#2001,.F.);
#2581=ORIENTED_EDGE('',*,*,#1997,.F.);
#2582=ORIENTED_EDGE('',*,*,#2002,.F.);
#2583=ORIENTED_EDGE('',*,*,#2003,.T.);
#2584=ORIENTED_EDGE('',*,*,#2004,.F.);
#2585=ORIENTED_EDGE('',*,*,#2003,.F.);
#2586=ORIENTED_EDGE('',*,*,#1916,.T.);
#2587=ORIENTED_EDGE('',*,*,#2005,.T.);
#2588=ORIENTED_EDGE('',*,*,#2006,.T.);
#2589=ORIENTED_EDGE('',*,*,#2007,.F.);
#2590=ORIENTED_EDGE('',*,*,#1893,.T.);
#2591=ORIENTED_EDGE('',*,*,#2008,.F.);
#2592=ORIENTED_EDGE('',*,*,#2009,.F.);
#2593=ORIENTED_EDGE('',*,*,#2010,.T.);
#2594=ORIENTED_EDGE('',*,*,#1944,.T.);
#2595=ORIENTED_EDGE('',*,*,#2011,.T.);
#2596=ORIENTED_EDGE('',*,*,#2009,.T.);
#2597=ORIENTED_EDGE('',*,*,#2012,.F.);
#2598=ORIENTED_EDGE('',*,*,#1921,.T.);
#2599=ORIENTED_EDGE('',*,*,#2013,.F.);
#2600=ORIENTED_EDGE('',*,*,#2014,.F.);
#2601=ORIENTED_EDGE('',*,*,#2015,.T.);
#2602=ORIENTED_EDGE('',*,*,#1972,.T.);
#2603=ORIENTED_EDGE('',*,*,#2016,.T.);
#2604=ORIENTED_EDGE('',*,*,#2014,.T.);
#2605=ORIENTED_EDGE('',*,*,#2017,.F.);
#2606=ORIENTED_EDGE('',*,*,#1949,.T.);
#2607=ORIENTED_EDGE('',*,*,#2018,.F.);
#2608=ORIENTED_EDGE('',*,*,#2019,.F.);
#2609=ORIENTED_EDGE('',*,*,#2020,.T.);
#2610=ORIENTED_EDGE('',*,*,#2000,.T.);
#2611=ORIENTED_EDGE('',*,*,#2021,.T.);
#2612=ORIENTED_EDGE('',*,*,#2019,.T.);
#2613=ORIENTED_EDGE('',*,*,#2022,.F.);
#2614=ORIENTED_EDGE('',*,*,#1977,.T.);
#2615=ORIENTED_EDGE('',*,*,#2023,.F.);
#2616=ORIENTED_EDGE('',*,*,#2006,.F.);
#2617=ORIENTED_EDGE('',*,*,#2024,.T.);
#2618=ORIENTED_EDGE('',*,*,#1892,.T.);
#2619=ORIENTED_EDGE('',*,*,#1896,.T.);
#2620=ORIENTED_EDGE('',*,*,#1899,.T.);
#2621=ORIENTED_EDGE('',*,*,#1902,.T.);
#2622=ORIENTED_EDGE('',*,*,#1905,.T.);
#2623=ORIENTED_EDGE('',*,*,#1908,.T.);
#2624=ORIENTED_EDGE('',*,*,#1911,.T.);
#2625=ORIENTED_EDGE('',*,*,#1914,.T.);
#2626=ORIENTED_EDGE('',*,*,#1917,.T.);
#2627=ORIENTED_EDGE('',*,*,#2007,.T.);
#2628=ORIENTED_EDGE('',*,*,#2023,.T.);
#2629=ORIENTED_EDGE('',*,*,#1976,.T.);
#2630=ORIENTED_EDGE('',*,*,#1980,.T.);
#2631=ORIENTED_EDGE('',*,*,#1983,.T.);
#2632=ORIENTED_EDGE('',*,*,#1986,.T.);
#2633=ORIENTED_EDGE('',*,*,#1989,.T.);
#2634=ORIENTED_EDGE('',*,*,#1992,.T.);
#2635=ORIENTED_EDGE('',*,*,#1995,.T.);
#2636=ORIENTED_EDGE('',*,*,#1998,.T.);
#2637=ORIENTED_EDGE('',*,*,#2001,.T.);
#2638=ORIENTED_EDGE('',*,*,#2022,.T.);
#2639=ORIENTED_EDGE('',*,*,#2018,.T.);
#2640=ORIENTED_EDGE('',*,*,#1948,.T.);
#2641=ORIENTED_EDGE('',*,*,#1952,.T.);
#2642=ORIENTED_EDGE('',*,*,#1955,.T.);
#2643=ORIENTED_EDGE('',*,*,#1958,.T.);
#2644=ORIENTED_EDGE('',*,*,#1961,.T.);
#2645=ORIENTED_EDGE('',*,*,#1964,.T.);
#2646=ORIENTED_EDGE('',*,*,#1967,.T.);
#2647=ORIENTED_EDGE('',*,*,#1970,.T.);
#2648=ORIENTED_EDGE('',*,*,#1973,.T.);
#2649=ORIENTED_EDGE('',*,*,#2017,.T.);
#2650=ORIENTED_EDGE('',*,*,#2013,.T.);
#2651=ORIENTED_EDGE('',*,*,#1920,.T.);
#2652=ORIENTED_EDGE('',*,*,#1924,.T.);
#2653=ORIENTED_EDGE('',*,*,#1927,.T.);
#2654=ORIENTED_EDGE('',*,*,#1930,.T.);
#2655=ORIENTED_EDGE('',*,*,#1933,.T.);
#2656=ORIENTED_EDGE('',*,*,#1936,.T.);
#2657=ORIENTED_EDGE('',*,*,#1939,.T.);
#2658=ORIENTED_EDGE('',*,*,#1942,.T.);
#2659=ORIENTED_EDGE('',*,*,#1945,.T.);
#2660=ORIENTED_EDGE('',*,*,#2012,.T.);
#2661=ORIENTED_EDGE('',*,*,#2008,.T.);
#2662=ORIENTED_EDGE('',*,*,#2004,.T.);
#2663=ORIENTED_EDGE('',*,*,#1890,.T.);
#2664=ORIENTED_EDGE('',*,*,#2010,.F.);
#2665=ORIENTED_EDGE('',*,*,#2011,.F.);
#2666=ORIENTED_EDGE('',*,*,#1943,.T.);
#2667=ORIENTED_EDGE('',*,*,#1940,.T.);
#2668=ORIENTED_EDGE('',*,*,#1937,.T.);
#2669=ORIENTED_EDGE('',*,*,#1934,.T.);
#2670=ORIENTED_EDGE('',*,*,#1931,.T.);
#2671=ORIENTED_EDGE('',*,*,#1928,.T.);
#2672=ORIENTED_EDGE('',*,*,#1925,.T.);
#2673=ORIENTED_EDGE('',*,*,#1922,.T.);
#2674=ORIENTED_EDGE('',*,*,#1918,.T.);
#2675=ORIENTED_EDGE('',*,*,#2015,.F.);
#2676=ORIENTED_EDGE('',*,*,#2016,.F.);
#2677=ORIENTED_EDGE('',*,*,#1971,.T.);
#2678=ORIENTED_EDGE('',*,*,#1968,.T.);
#2679=ORIENTED_EDGE('',*,*,#1965,.T.);
#2680=ORIENTED_EDGE('',*,*,#1962,.T.);
#2681=ORIENTED_EDGE('',*,*,#1959,.T.);
#2682=ORIENTED_EDGE('',*,*,#1956,.T.);
#2683=ORIENTED_EDGE('',*,*,#1953,.T.);
#2684=ORIENTED_EDGE('',*,*,#1950,.T.);
#2685=ORIENTED_EDGE('',*,*,#1946,.T.);
#2686=ORIENTED_EDGE('',*,*,#2020,.F.);
#2687=ORIENTED_EDGE('',*,*,#2021,.F.);
#2688=ORIENTED_EDGE('',*,*,#1999,.T.);
#2689=ORIENTED_EDGE('',*,*,#1996,.T.);
#2690=ORIENTED_EDGE('',*,*,#1993,.T.);
#2691=ORIENTED_EDGE('',*,*,#1990,.T.);
#2692=ORIENTED_EDGE('',*,*,#1987,.T.);
#2693=ORIENTED_EDGE('',*,*,#1984,.T.);
#2694=ORIENTED_EDGE('',*,*,#1981,.T.);
#2695=ORIENTED_EDGE('',*,*,#1978,.T.);
#2696=ORIENTED_EDGE('',*,*,#1974,.T.);
#2697=ORIENTED_EDGE('',*,*,#2024,.F.);
#2698=ORIENTED_EDGE('',*,*,#2005,.F.);
#2699=ORIENTED_EDGE('',*,*,#1915,.T.);
#2700=ORIENTED_EDGE('',*,*,#1912,.T.);
#2701=ORIENTED_EDGE('',*,*,#1909,.T.);
#2702=ORIENTED_EDGE('',*,*,#1906,.T.);
#2703=ORIENTED_EDGE('',*,*,#1903,.T.);
#2704=ORIENTED_EDGE('',*,*,#1900,.T.);
#2705=ORIENTED_EDGE('',*,*,#1897,.T.);
#2706=ORIENTED_EDGE('',*,*,#1894,.T.);
#2707=ORIENTED_EDGE('',*,*,#2002,.T.);
#3106=CYLINDRICAL_SURFACE('',#3595,0.21);
#3186=ADVANCED_FACE('',(#393),#242,.F.);
#3187=ADVANCED_FACE('',(#394),#243,.F.);
#3188=ADVANCED_FACE('',(#395),#244,.F.);
#3189=ADVANCED_FACE('',(#396),#245,.F.);
#3190=ADVANCED_FACE('',(#397),#246,.F.);
#3191=ADVANCED_FACE('',(#398),#247,.F.);
#3192=ADVANCED_FACE('',(#399),#248,.F.);
#3193=ADVANCED_FACE('',(#400),#249,.F.);
#3194=ADVANCED_FACE('',(#401),#250,.F.);
#3195=ADVANCED_FACE('',(#402),#251,.F.);
#3196=ADVANCED_FACE('',(#403),#252,.F.);
#3197=ADVANCED_FACE('',(#404),#253,.F.);
#3198=ADVANCED_FACE('',(#405),#254,.F.);
#3199=ADVANCED_FACE('',(#406),#255,.F.);
#3200=ADVANCED_FACE('',(#407),#256,.F.);
#3201=ADVANCED_FACE('',(#408),#257,.F.);
#3202=ADVANCED_FACE('',(#409),#258,.F.);
#3203=ADVANCED_FACE('',(#410),#259,.F.);
#3204=ADVANCED_FACE('',(#411),#260,.F.);
#3205=ADVANCED_FACE('',(#412),#261,.F.);
#3206=ADVANCED_FACE('',(#413),#262,.F.);
#3207=ADVANCED_FACE('',(#414),#263,.F.);
#3208=ADVANCED_FACE('',(#415),#264,.F.);
#3209=ADVANCED_FACE('',(#416),#265,.F.);
#3210=ADVANCED_FACE('',(#417),#266,.F.);
#3211=ADVANCED_FACE('',(#418),#267,.F.);
#3212=ADVANCED_FACE('',(#419),#268,.F.);
#3213=ADVANCED_FACE('',(#420),#269,.F.);
#3214=ADVANCED_FACE('',(#421),#270,.F.);
#3215=ADVANCED_FACE('',(#422),#271,.F.);
#3216=ADVANCED_FACE('',(#423),#272,.F.);
#3217=ADVANCED_FACE('',(#424),#273,.F.);
#3218=ADVANCED_FACE('',(#425),#274,.F.);
#3219=ADVANCED_FACE('',(#426),#275,.F.);
#3220=ADVANCED_FACE('',(#427),#276,.F.);
#3221=ADVANCED_FACE('',(#428),#277,.F.);
#3222=ADVANCED_FACE('',(#429),#3106,.F.);
#3223=ADVANCED_FACE('',(#430),#278,.T.);
#3224=ADVANCED_FACE('',(#431),#279,.T.);
#3225=ADVANCED_FACE('',(#432),#280,.T.);
#3226=ADVANCED_FACE('',(#433),#281,.T.);
#3227=ADVANCED_FACE('',(#434),#282,.T.);
#3228=ADVANCED_FACE('',(#435),#283,.T.);
#3229=ADVANCED_FACE('',(#436),#284,.T.);
#3230=ADVANCED_FACE('',(#437),#285,.T.);
#3231=ADVANCED_FACE('',(#438,#183),#286,.T.);
#3232=ADVANCED_FACE('',(#439,#184),#287,.F.);
#3326=CLOSED_SHELL('',(#3186,#3187,#3188,#3189,#3190,#3191,#3192,#3193,
#3194,#3195,#3196,#3197,#3198,#3199,#3200,#3201,#3202,#3203,#3204,#3205,
#3206,#3207,#3208,#3209,#3210,#3211,#3212,#3213,#3214,#3215,#3216,#3217,
#3218,#3219,#3220,#3221,#3222,#3223,#3224,#3225,#3226,#3227,#3228,#3229,
#3230,#3231,#3232));
#3558=AXIS2_PLACEMENT_3D('',#4987,#4045,#4046);
#3559=AXIS2_PLACEMENT_3D('',#4988,#4047,#4048);
#3560=AXIS2_PLACEMENT_3D('',#4997,#4053,#4054);
#3561=AXIS2_PLACEMENT_3D('',#5003,#4058,#4059);
#3562=AXIS2_PLACEMENT_3D('',#5009,#4063,#4064);
#3563=AXIS2_PLACEMENT_3D('',#5015,#4068,#4069);
#3564=AXIS2_PLACEMENT_3D('',#5021,#4073,#4074);
#3565=AXIS2_PLACEMENT_3D('',#5027,#4078,#4079);
#3566=AXIS2_PLACEMENT_3D('',#5033,#4083,#4084);
#3567=AXIS2_PLACEMENT_3D('',#5039,#4088,#4089);
#3568=AXIS2_PLACEMENT_3D('',#5045,#4093,#4094);
#3569=AXIS2_PLACEMENT_3D('',#5054,#4099,#4100);
#3570=AXIS2_PLACEMENT_3D('',#5060,#4104,#4105);
#3571=AXIS2_PLACEMENT_3D('',#5066,#4109,#4110);
#3572=AXIS2_PLACEMENT_3D('',#5072,#4114,#4115);
#3573=AXIS2_PLACEMENT_3D('',#5078,#4119,#4120);
#3574=AXIS2_PLACEMENT_3D('',#5084,#4124,#4125);
#3575=AXIS2_PLACEMENT_3D('',#5090,#4129,#4130);
#3576=AXIS2_PLACEMENT_3D('',#5096,#4134,#4135);
#3577=AXIS2_PLACEMENT_3D('',#5102,#4139,#4140);
#3578=AXIS2_PLACEMENT_3D('',#5111,#4145,#4146);
#3579=AXIS2_PLACEMENT_3D('',#5117,#4150,#4151);
#3580=AXIS2_PLACEMENT_3D('',#5123,#4155,#4156);
#3581=AXIS2_PLACEMENT_3D('',#5129,#4160,#4161);
#3582=AXIS2_PLACEMENT_3D('',#5135,#4165,#4166);
#3583=AXIS2_PLACEMENT_3D('',#5141,#4170,#4171);
#3584=AXIS2_PLACEMENT_3D('',#5147,#4175,#4176);
#3585=AXIS2_PLACEMENT_3D('',#5153,#4180,#4181);
#3586=AXIS2_PLACEMENT_3D('',#5159,#4185,#4186);
#3587=AXIS2_PLACEMENT_3D('',#5168,#4191,#4192);
#3588=AXIS2_PLACEMENT_3D('',#5174,#4196,#4197);
#3589=AXIS2_PLACEMENT_3D('',#5180,#4201,#4202);
#3590=AXIS2_PLACEMENT_3D('',#5186,#4206,#4207);
#3591=AXIS2_PLACEMENT_3D('',#5192,#4211,#4212);
#3592=AXIS2_PLACEMENT_3D('',#5198,#4216,#4217);
#3593=AXIS2_PLACEMENT_3D('',#5204,#4221,#4222);
#3594=AXIS2_PLACEMENT_3D('',#5210,#4226,#4227);
#3595=AXIS2_PLACEMENT_3D('',#5216,#4231,#4232);
#3596=AXIS2_PLACEMENT_3D('',#5218,#4233,#4234);
#3597=AXIS2_PLACEMENT_3D('',#5221,#4236,#4237);
#3598=AXIS2_PLACEMENT_3D('',#5222,#4238,#4239);
#3599=AXIS2_PLACEMENT_3D('',#5228,#4243,#4244);
#3600=AXIS2_PLACEMENT_3D('',#5234,#4248,#4249);
#3601=AXIS2_PLACEMENT_3D('',#5237,#4252,#4253);
#3602=AXIS2_PLACEMENT_3D('',#5243,#4257,#4258);
#3603=AXIS2_PLACEMENT_3D('',#5246,#4261,#4262);
#3604=AXIS2_PLACEMENT_3D('',#5252,#4266,#4267);
#3605=AXIS2_PLACEMENT_3D('',#5255,#4270,#4271);
#3606=AXIS2_PLACEMENT_3D('',#5258,#4274,#4275);
#3607=AXIS2_PLACEMENT_3D('',#5259,#4276,#4277);
#4045=DIRECTION('axis',(0.,0.,1.));
#4046=DIRECTION('refdir',(1.,0.,0.));
#4047=DIRECTION('center_axis',(0.,0.,-1.));
#4048=DIRECTION('ref_axis',(0.,1.,0.));
#4049=DIRECTION('',(0.,1.,0.));
#4050=DIRECTION('',(1.,0.,0.));
#4051=DIRECTION('',(0.,-1.,0.));
#4052=DIRECTION('',(1.,0.,0.));
#4053=DIRECTION('center_axis',(0.,1.,-8.88178419700125E-16));
#4054=DIRECTION('ref_axis',(0.,8.88178419700125E-16,1.));
#4055=DIRECTION('',(0.,8.88178419700125E-16,1.));
#4056=DIRECTION('',(1.,0.,0.));
#4057=DIRECTION('',(0.,-8.88178419700125E-16,-1.));
#4058=DIRECTION('center_axis',(0.,-7.40148683083439E-16,-1.));
#4059=DIRECTION('ref_axis',(0.,1.,-7.40148683083439E-16));
#4060=DIRECTION('',(0.,1.,-7.40148683083439E-16));
#4061=DIRECTION('',(1.,0.,0.));
#4062=DIRECTION('',(0.,-1.,7.40148683083439E-16));
#4063=DIRECTION('center_axis',(0.,-0.707106781186547,-0.707106781186548));
#4064=DIRECTION('ref_axis',(0.,0.707106781186548,-0.707106781186547));
#4065=DIRECTION('',(0.,0.707106781186548,-0.707106781186547));
#4066=DIRECTION('',(1.,0.,0.));
#4067=DIRECTION('',(0.,-0.707106781186548,0.707106781186547));
#4068=DIRECTION('center_axis',(0.,-1.,2.77555756156289E-16));
#4069=DIRECTION('ref_axis',(0.,-2.77555756156289E-16,-1.));
#4070=DIRECTION('',(0.,-2.77555756156289E-16,-1.));
#4071=DIRECTION('',(1.,0.,0.));
#4072=DIRECTION('',(0.,2.77555756156289E-16,1.));
#4073=DIRECTION('center_axis',(0.,-0.707106781186547,0.707106781186548));
#4074=DIRECTION('ref_axis',(0.,-0.707106781186548,-0.707106781186547));
#4075=DIRECTION('',(0.,-0.707106781186548,-0.707106781186547));
#4076=DIRECTION('',(1.,0.,0.));
#4077=DIRECTION('',(0.,0.707106781186548,0.707106781186547));
#4078=DIRECTION('center_axis',(0.,7.40148683083438E-16,1.));
#4079=DIRECTION('ref_axis',(0.,-1.,7.40148683083438E-16));
#4080=DIRECTION('',(0.,-1.,7.40148683083438E-16));
#4081=DIRECTION('',(1.,0.,0.));
#4082=DIRECTION('',(0.,1.,-7.40148683083438E-16));
#4083=DIRECTION('center_axis',(0.,1.,-4.44089209850063E-16));
#4084=DIRECTION('ref_axis',(0.,4.44089209850063E-16,1.));
#4085=DIRECTION('',(0.,4.44089209850063E-16,1.));
#4086=DIRECTION('',(1.,0.,0.));
#4087=DIRECTION('',(0.,-4.44089209850063E-16,-1.));
#4088=DIRECTION('center_axis',(0.,2.41352831440251E-16,1.));
#4089=DIRECTION('ref_axis',(0.,-1.,2.41352831440251E-16));
#4090=DIRECTION('',(0.,-1.,2.41352831440251E-16));
#4091=DIRECTION('',(-1.,0.,0.));
#4092=DIRECTION('',(0.,1.,-2.41352831440251E-16));
#4093=DIRECTION('center_axis',(0.,-1.,2.41352831440251E-16));
#4094=DIRECTION('ref_axis',(0.,-2.41352831440251E-16,-1.));
#4095=DIRECTION('',(0.,-2.41352831440251E-16,-1.));
#4096=DIRECTION('',(1.,0.,0.));
#4097=DIRECTION('',(0.,2.41352831440251E-16,1.));
#4098=DIRECTION('',(1.,0.,0.));
#4099=DIRECTION('center_axis',(0.,0.,-1.));
#4100=DIRECTION('ref_axis',(0.,1.,0.));
#4101=DIRECTION('',(0.,1.,0.));
#4102=DIRECTION('',(1.,0.,0.));
#4103=DIRECTION('',(0.,-1.,0.));
#4104=DIRECTION('center_axis',(0.,-1.,0.));
#4105=DIRECTION('ref_axis',(0.,0.,-1.));
#4106=DIRECTION('',(0.,0.,-1.));
#4107=DIRECTION('',(1.,0.,0.));
#4108=DIRECTION('',(0.,0.,1.));
#4109=DIRECTION('center_axis',(0.,-0.707106781186547,0.707106781186548));
#4110=DIRECTION('ref_axis',(0.,-0.707106781186548,-0.707106781186547));
#4111=DIRECTION('',(0.,-0.707106781186548,-0.707106781186547));
#4112=DIRECTION('',(1.,0.,0.));
#4113=DIRECTION('',(0.,0.707106781186548,0.707106781186547));
#4114=DIRECTION('center_axis',(0.,0.,1.));
#4115=DIRECTION('ref_axis',(0.,-1.,0.));
#4116=DIRECTION('',(0.,-1.,0.));
#4117=DIRECTION('',(1.,0.,0.));
#4118=DIRECTION('',(0.,1.,0.));
#4119=DIRECTION('center_axis',(0.,0.707106781186548,0.707106781186547));
#4120=DIRECTION('ref_axis',(0.,-0.707106781186547,0.707106781186548));
#4121=DIRECTION('',(0.,-0.707106781186547,0.707106781186548));
#4122=DIRECTION('',(1.,0.,0.));
#4123=DIRECTION('',(0.,0.707106781186547,-0.707106781186548));
#4124=DIRECTION('center_axis',(0.,1.,0.));
#4125=DIRECTION('ref_axis',(0.,0.,1.));
#4126=DIRECTION('',(0.,0.,1.));
#4127=DIRECTION('',(1.,0.,0.));
#4128=DIRECTION('',(0.,0.,-1.));
#4129=DIRECTION('center_axis',(0.,0.,-1.));
#4130=DIRECTION('ref_axis',(0.,1.,0.));
#4131=DIRECTION('',(0.,1.,0.));
#4132=DIRECTION('',(1.,0.,0.));
#4133=DIRECTION('',(0.,-1.,0.));
#4134=DIRECTION('center_axis',(0.,1.,-2.41352831440251E-16));
#4135=DIRECTION('ref_axis',(0.,2.41352831440251E-16,1.));
#4136=DIRECTION('',(0.,2.41352831440251E-16,1.));
#4137=DIRECTION('',(-1.,0.,0.));
#4138=DIRECTION('',(0.,-2.41352831440251E-16,-1.));
#4139=DIRECTION('center_axis',(0.,0.,1.));
#4140=DIRECTION('ref_axis',(0.,-1.,0.));
#4141=DIRECTION('',(0.,-1.,0.));
#4142=DIRECTION('',(1.,0.,0.));
#4143=DIRECTION('',(0.,1.,0.));
#4144=DIRECTION('',(1.,0.,0.));
#4145=DIRECTION('center_axis',(0.,-1.,0.));
#4146=DIRECTION('ref_axis',(0.,0.,-1.));
#4147=DIRECTION('',(0.,0.,-1.));
#4148=DIRECTION('',(1.,0.,0.));
#4149=DIRECTION('',(0.,0.,1.));
#4150=DIRECTION('center_axis',(0.,0.,1.));
#4151=DIRECTION('ref_axis',(0.,-1.,0.));
#4152=DIRECTION('',(0.,-1.,0.));
#4153=DIRECTION('',(1.,0.,0.));
#4154=DIRECTION('',(0.,1.,0.));
#4155=DIRECTION('center_axis',(0.,0.707106781186548,0.707106781186548));
#4156=DIRECTION('ref_axis',(0.,-0.707106781186548,0.707106781186548));
#4157=DIRECTION('',(0.,-0.707106781186548,0.707106781186548));
#4158=DIRECTION('',(1.,0.,0.));
#4159=DIRECTION('',(0.,0.707106781186548,-0.707106781186548));
#4160=DIRECTION('center_axis',(0.,1.,0.));
#4161=DIRECTION('ref_axis',(0.,0.,1.));
#4162=DIRECTION('',(0.,0.,1.));
#4163=DIRECTION('',(1.,0.,0.));
#4164=DIRECTION('',(0.,0.,-1.));
#4165=DIRECTION('center_axis',(0.,0.707106781186548,-0.707106781186547));
#4166=DIRECTION('ref_axis',(0.,0.707106781186547,0.707106781186548));
#4167=DIRECTION('',(0.,0.707106781186547,0.707106781186548));
#4168=DIRECTION('',(1.,0.,0.));
#4169=DIRECTION('',(0.,-0.707106781186547,-0.707106781186548));
#4170=DIRECTION('center_axis',(0.,-7.40148683083438E-16,-1.));
#4171=DIRECTION('ref_axis',(0.,1.,-7.40148683083438E-16));
#4172=DIRECTION('',(0.,1.,-7.40148683083438E-16));
#4173=DIRECTION('',(1.,0.,0.));
#4174=DIRECTION('',(0.,-1.,7.40148683083438E-16));
#4175=DIRECTION('center_axis',(0.,-1.,0.));
#4176=DIRECTION('ref_axis',(0.,0.,-1.));
#4177=DIRECTION('',(0.,0.,-1.));
#4178=DIRECTION('',(1.,0.,0.));
#4179=DIRECTION('',(0.,0.,1.));
#4180=DIRECTION('center_axis',(0.,0.,-1.));
#4181=DIRECTION('ref_axis',(0.,1.,0.));
#4182=DIRECTION('',(0.,1.,0.));
#4183=DIRECTION('',(-1.,0.,0.));
#4184=DIRECTION('',(0.,-1.,0.));
#4185=DIRECTION('center_axis',(0.,1.,0.));
#4186=DIRECTION('ref_axis',(0.,0.,1.));
#4187=DIRECTION('',(0.,0.,1.));
#4188=DIRECTION('',(1.,0.,0.));
#4189=DIRECTION('',(0.,0.,-1.));
#4190=DIRECTION('',(1.,0.,0.));
#4191=DIRECTION('center_axis',(0.,0.,1.));
#4192=DIRECTION('ref_axis',(0.,-1.,0.));
#4193=DIRECTION('',(0.,-1.,0.));
#4194=DIRECTION('',(1.,0.,0.));
#4195=DIRECTION('',(0.,1.,0.));
#4196=DIRECTION('center_axis',(0.,1.,0.));
#4197=DIRECTION('ref_axis',(0.,0.,1.));
#4198=DIRECTION('',(0.,0.,1.));
#4199=DIRECTION('',(1.,0.,0.));
#4200=DIRECTION('',(0.,0.,-1.));
#4201=DIRECTION('center_axis',(0.,0.707106781186547,-0.707106781186548));
#4202=DIRECTION('ref_axis',(0.,0.707106781186548,0.707106781186547));
#4203=DIRECTION('',(0.,0.707106781186548,0.707106781186547));
#4204=DIRECTION('',(1.,0.,0.));
#4205=DIRECTION('',(0.,-0.707106781186548,-0.707106781186547));
#4206=DIRECTION('center_axis',(0.,0.,-1.));
#4207=DIRECTION('ref_axis',(0.,1.,0.));
#4208=DIRECTION('',(0.,1.,0.));
#4209=DIRECTION('',(1.,0.,0.));
#4210=DIRECTION('',(0.,-1.,0.));
#4211=DIRECTION('center_axis',(0.,-0.707106781186547,-0.707106781186548));
#4212=DIRECTION('ref_axis',(0.,0.707106781186548,-0.707106781186547));
#4213=DIRECTION('',(0.,0.707106781186548,-0.707106781186547));
#4214=DIRECTION('',(1.,0.,0.));
#4215=DIRECTION('',(0.,-0.707106781186548,0.707106781186547));
#4216=DIRECTION('center_axis',(0.,-1.,0.));
#4217=DIRECTION('ref_axis',(0.,0.,-1.));
#4218=DIRECTION('',(0.,0.,-1.));
#4219=DIRECTION('',(1.,0.,0.));
#4220=DIRECTION('',(0.,0.,1.));
#4221=DIRECTION('center_axis',(0.,0.,1.));
#4222=DIRECTION('ref_axis',(0.,-1.,0.));
#4223=DIRECTION('',(0.,-1.,0.));
#4224=DIRECTION('',(1.,0.,0.));
#4225=DIRECTION('',(0.,1.,0.));
#4226=DIRECTION('center_axis',(0.,-1.,0.));
#4227=DIRECTION('ref_axis',(0.,0.,-1.));
#4228=DIRECTION('',(0.,0.,-1.));
#4229=DIRECTION('',(-1.,0.,0.));
#4230=DIRECTION('',(0.,0.,1.));
#4231=DIRECTION('center_axis',(1.,0.,0.));
#4232=DIRECTION('ref_axis',(0.,0.,-1.));
#4233=DIRECTION('center_axis',(1.,0.,0.));
#4234=DIRECTION('ref_axis',(0.,0.,-1.));
#4235=DIRECTION('',(1.,0.,0.));
#4236=DIRECTION('center_axis',(-1.,0.,0.));
#4237=DIRECTION('ref_axis',(0.,0.,-1.));
#4238=DIRECTION('center_axis',(0.,1.,0.));
#4239=DIRECTION('ref_axis',(0.,0.,1.));
#4240=DIRECTION('',(0.,0.,1.));
#4241=DIRECTION('',(1.,0.,0.));
#4242=DIRECTION('',(0.,0.,1.));
#4243=DIRECTION('center_axis',(0.,1.,0.));
#4244=DIRECTION('ref_axis',(0.,0.,1.));
#4245=DIRECTION('',(0.,0.,1.));
#4246=DIRECTION('',(1.,0.,0.));
#4247=DIRECTION('',(0.,0.,1.));
#4248=DIRECTION('center_axis',(0.,0.,-1.));
#4249=DIRECTION('ref_axis',(0.,1.,0.));
#4250=DIRECTION('',(0.,1.,0.));
#4251=DIRECTION('',(0.,1.,0.));
#4252=DIRECTION('center_axis',(0.,0.,-1.));
#4253=DIRECTION('ref_axis',(0.,1.,0.));
#4254=DIRECTION('',(0.,1.,0.));
#4255=DIRECTION('',(1.,0.,0.));
#4256=DIRECTION('',(0.,1.,0.));
#4257=DIRECTION('center_axis',(0.,-1.,0.));
#4258=DIRECTION('ref_axis',(0.,0.,-1.));
#4259=DIRECTION('',(0.,0.,-1.));
#4260=DIRECTION('',(0.,0.,-1.));
#4261=DIRECTION('center_axis',(0.,-1.,0.));
#4262=DIRECTION('ref_axis',(0.,0.,-1.));
#4263=DIRECTION('',(0.,0.,-1.));
#4264=DIRECTION('',(1.,0.,0.));
#4265=DIRECTION('',(0.,0.,-1.));
#4266=DIRECTION('center_axis',(0.,0.,1.));
#4267=DIRECTION('ref_axis',(0.,-1.,0.));
#4268=DIRECTION('',(0.,-1.,0.));
#4269=DIRECTION('',(0.,-1.,0.));
#4270=DIRECTION('center_axis',(0.,0.,1.));
#4271=DIRECTION('ref_axis',(0.,-1.,0.));
#4272=DIRECTION('',(0.,-1.,0.));
#4273=DIRECTION('',(0.,-1.,0.));
#4274=DIRECTION('center_axis',(1.,0.,0.));
#4275=DIRECTION('ref_axis',(0.,0.,-1.));
#4276=DIRECTION('center_axis',(1.,0.,0.));
#4277=DIRECTION('ref_axis',(0.,0.,-1.));
#4987=CARTESIAN_POINT('',(0.,0.,0.));
#4988=CARTESIAN_POINT('Origin',(-0.1,0.82,-0.3));
#4989=CARTESIAN_POINT('',(0.,0.82,-0.3));
#4990=CARTESIAN_POINT('',(0.,1.,-0.3));
#4991=CARTESIAN_POINT('',(0.,0.41,-0.3));
#4992=CARTESIAN_POINT('',(10.,0.82,-0.3));
#4993=CARTESIAN_POINT('',(-0.1,0.82,-0.3));
#4994=CARTESIAN_POINT('',(10.,1.,-0.3));
#4995=CARTESIAN_POINT('',(10.,0.41,-0.3));
#4996=CARTESIAN_POINT('',(-0.05,1.,-0.3));
#4997=CARTESIAN_POINT('Origin',(-0.1,0.82,-0.55));
#4998=CARTESIAN_POINT('',(0.,0.82,-0.55));
#4999=CARTESIAN_POINT('',(0.,0.82,-0.275));
#5000=CARTESIAN_POINT('',(10.,0.82,-0.55));
#5001=CARTESIAN_POINT('',(-0.1,0.82,-0.55));
#5002=CARTESIAN_POINT('',(10.,0.82,-0.275));
#5003=CARTESIAN_POINT('Origin',(-0.1,0.67,-0.55));
#5004=CARTESIAN_POINT('',(0.,0.67,-0.55));
#5005=CARTESIAN_POINT('',(0.,0.335,-0.55));
#5006=CARTESIAN_POINT('',(10.,0.67,-0.55));
#5007=CARTESIAN_POINT('',(-0.1,0.67,-0.55));
#5008=CARTESIAN_POINT('',(10.,0.335,-0.55));
#5009=CARTESIAN_POINT('Origin',(-0.1,0.42,-0.3));
#5010=CARTESIAN_POINT('',(0.,0.42,-0.3));
#5011=CARTESIAN_POINT('',(0.,0.24,-0.12));
#5012=CARTESIAN_POINT('',(10.,0.42,-0.3));
#5013=CARTESIAN_POINT('',(-0.1,0.42,-0.3));
#5014=CARTESIAN_POINT('',(10.,0.24,-0.12));
#5015=CARTESIAN_POINT('Origin',(-0.1,0.42,0.3));
#5016=CARTESIAN_POINT('',(0.,0.42,0.3));
#5017=CARTESIAN_POINT('',(0.,0.42,0.15));
#5018=CARTESIAN_POINT('',(10.,0.42,0.3));
#5019=CARTESIAN_POINT('',(-0.1,0.42,0.3));
#5020=CARTESIAN_POINT('',(10.,0.42,0.15));
#5021=CARTESIAN_POINT('Origin',(-0.1,0.67,0.55));
#5022=CARTESIAN_POINT('',(0.,0.67,0.55));
#5023=CARTESIAN_POINT('',(6.93889390390723E-18,0.365,0.245));
#5024=CARTESIAN_POINT('',(10.,0.67,0.55));
#5025=CARTESIAN_POINT('',(-0.1,0.67,0.55));
#5026=CARTESIAN_POINT('',(10.,0.365,0.245));
#5027=CARTESIAN_POINT('Origin',(-0.1,0.82,0.55));
#5028=CARTESIAN_POINT('',(0.,0.82,0.55));
#5029=CARTESIAN_POINT('',(0.,0.41,0.55));
#5030=CARTESIAN_POINT('',(10.,0.82,0.55));
#5031=CARTESIAN_POINT('',(-0.1,0.82,0.55));
#5032=CARTESIAN_POINT('',(10.,0.41,0.55));
#5033=CARTESIAN_POINT('Origin',(-0.1,0.82,0.3));
#5034=CARTESIAN_POINT('',(0.,0.82,0.3));
#5035=CARTESIAN_POINT('',(0.,0.82,0.15));
#5036=CARTESIAN_POINT('',(10.,0.82,0.3));
#5037=CARTESIAN_POINT('',(-0.1,0.82,0.3));
#5038=CARTESIAN_POINT('',(10.,0.82,0.15));
#5039=CARTESIAN_POINT('Origin',(-0.1,1.05,0.3));
#5040=CARTESIAN_POINT('',(0.,1.,0.3));
#5041=CARTESIAN_POINT('',(0.,0.525,0.3));
#5042=CARTESIAN_POINT('',(10.,1.,0.3));
#5043=CARTESIAN_POINT('',(-0.05,1.,0.3));
#5044=CARTESIAN_POINT('',(10.,0.525,0.3));
#5045=CARTESIAN_POINT('Origin',(-0.1,-0.3,-0.82));
#5046=CARTESIAN_POINT('',(0.,-0.3,-0.82));
#5047=CARTESIAN_POINT('',(0.,-0.3,-1.));
#5048=CARTESIAN_POINT('',(0.,-0.3,-0.41));
#5049=CARTESIAN_POINT('',(10.,-0.3,-0.82));
#5050=CARTESIAN_POINT('',(-0.1,-0.3,-0.82));
#5051=CARTESIAN_POINT('',(10.,-0.3,-1.));
#5052=CARTESIAN_POINT('',(10.,-0.3,-0.41));
#5053=CARTESIAN_POINT('',(-0.05,-0.3,-1.));
#5054=CARTESIAN_POINT('Origin',(-0.1,-0.55,-0.82));
#5055=CARTESIAN_POINT('',(0.,-0.55,-0.82));
#5056=CARTESIAN_POINT('',(0.,-0.275,-0.82));
#5057=CARTESIAN_POINT('',(10.,-0.55,-0.82));
#5058=CARTESIAN_POINT('',(-0.1,-0.55,-0.82));
#5059=CARTESIAN_POINT('',(10.,-0.275,-0.82));
#5060=CARTESIAN_POINT('Origin',(-0.1,-0.55,-0.67));
#5061=CARTESIAN_POINT('',(0.,-0.55,-0.67));
#5062=CARTESIAN_POINT('',(0.,-0.55,-0.335));
#5063=CARTESIAN_POINT('',(10.,-0.55,-0.67));
#5064=CARTESIAN_POINT('',(-0.1,-0.55,-0.67));
#5065=CARTESIAN_POINT('',(10.,-0.55,-0.335));
#5066=CARTESIAN_POINT('Origin',(-0.1,-0.3,-0.42));
#5067=CARTESIAN_POINT('',(0.,-0.3,-0.42));
#5068=CARTESIAN_POINT('',(0.,-0.12,-0.24));
#5069=CARTESIAN_POINT('',(10.,-0.3,-0.42));
#5070=CARTESIAN_POINT('',(-0.1,-0.3,-0.42));
#5071=CARTESIAN_POINT('',(10.,-0.12,-0.24));
#5072=CARTESIAN_POINT('Origin',(-0.1,0.3,-0.42));
#5073=CARTESIAN_POINT('',(0.,0.3,-0.42));
#5074=CARTESIAN_POINT('',(0.,0.15,-0.42));
#5075=CARTESIAN_POINT('',(10.,0.3,-0.42));
#5076=CARTESIAN_POINT('',(-0.1,0.3,-0.42));
#5077=CARTESIAN_POINT('',(10.,0.15,-0.42));
#5078=CARTESIAN_POINT('Origin',(-0.1,0.55,-0.67));
#5079=CARTESIAN_POINT('',(0.,0.55,-0.67));
#5080=CARTESIAN_POINT('',(0.,0.245,-0.365));
#5081=CARTESIAN_POINT('',(10.,0.55,-0.67));
#5082=CARTESIAN_POINT('',(-0.1,0.55,-0.67));
#5083=CARTESIAN_POINT('',(10.,0.245,-0.365));
#5084=CARTESIAN_POINT('Origin',(-0.1,0.55,-0.82));
#5085=CARTESIAN_POINT('',(0.,0.55,-0.82));
#5086=CARTESIAN_POINT('',(0.,0.55,-0.41));
#5087=CARTESIAN_POINT('',(10.,0.55,-0.82));
#5088=CARTESIAN_POINT('',(-0.1,0.55,-0.82));
#5089=CARTESIAN_POINT('',(10.,0.55,-0.41));
#5090=CARTESIAN_POINT('Origin',(-0.1,0.3,-0.82));
#5091=CARTESIAN_POINT('',(0.,0.3,-0.82));
#5092=CARTESIAN_POINT('',(0.,0.15,-0.82));
#5093=CARTESIAN_POINT('',(10.,0.3,-0.82));
#5094=CARTESIAN_POINT('',(-0.1,0.3,-0.82));
#5095=CARTESIAN_POINT('',(10.,0.15,-0.82));
#5096=CARTESIAN_POINT('Origin',(-0.1,0.3,-1.05));
#5097=CARTESIAN_POINT('',(0.,0.3,-1.));
#5098=CARTESIAN_POINT('',(0.,0.3,-0.525));
#5099=CARTESIAN_POINT('',(10.,0.3,-1.));
#5100=CARTESIAN_POINT('',(-0.05,0.3,-1.));
#5101=CARTESIAN_POINT('',(10.,0.3,-0.525));
#5102=CARTESIAN_POINT('Origin',(-0.1,-0.82,0.3));
#5103=CARTESIAN_POINT('',(0.,-0.82,0.3));
#5104=CARTESIAN_POINT('',(0.,-1.,0.3));
#5105=CARTESIAN_POINT('',(0.,-0.41,0.3));
#5106=CARTESIAN_POINT('',(10.,-0.82,0.3));
#5107=CARTESIAN_POINT('',(-0.1,-0.82,0.3));
#5108=CARTESIAN_POINT('',(10.,-1.,0.3));
#5109=CARTESIAN_POINT('',(10.,-0.41,0.3));
#5110=CARTESIAN_POINT('',(-0.05,-1.,0.3));
#5111=CARTESIAN_POINT('Origin',(-0.1,-0.82,0.55));
#5112=CARTESIAN_POINT('',(0.,-0.82,0.55));
#5113=CARTESIAN_POINT('',(0.,-0.82,0.275));
#5114=CARTESIAN_POINT('',(10.,-0.82,0.55));
#5115=CARTESIAN_POINT('',(-0.1,-0.82,0.55));
#5116=CARTESIAN_POINT('',(10.,-0.82,0.275));
#5117=CARTESIAN_POINT('Origin',(-0.1,-0.67,0.55));
#5118=CARTESIAN_POINT('',(0.,-0.67,0.55));
#5119=CARTESIAN_POINT('',(0.,-0.335,0.55));
#5120=CARTESIAN_POINT('',(10.,-0.67,0.55));
#5121=CARTESIAN_POINT('',(-0.1,-0.67,0.55));
#5122=CARTESIAN_POINT('',(10.,-0.335,0.55));
#5123=CARTESIAN_POINT('Origin',(-0.1,-0.42,0.3));
#5124=CARTESIAN_POINT('',(0.,-0.42,0.3));
#5125=CARTESIAN_POINT('',(-6.93889390390723E-18,-0.24,0.12));
#5126=CARTESIAN_POINT('',(10.,-0.42,0.3));
#5127=CARTESIAN_POINT('',(-0.1,-0.42,0.3));
#5128=CARTESIAN_POINT('',(10.,-0.24,0.12));
#5129=CARTESIAN_POINT('Origin',(-0.1,-0.42,-0.3));
#5130=CARTESIAN_POINT('',(0.,-0.42,-0.3));
#5131=CARTESIAN_POINT('',(0.,-0.42,-0.15));
#5132=CARTESIAN_POINT('',(10.,-0.42,-0.3));
#5133=CARTESIAN_POINT('',(-0.1,-0.42,-0.3));
#5134=CARTESIAN_POINT('',(10.,-0.42,-0.15));
#5135=CARTESIAN_POINT('Origin',(-0.1,-0.67,-0.55));
#5136=CARTESIAN_POINT('',(0.,-0.67,-0.55));
#5137=CARTESIAN_POINT('',(0.,-0.365,-0.245));
#5138=CARTESIAN_POINT('',(10.,-0.67,-0.55));
#5139=CARTESIAN_POINT('',(-0.1,-0.67,-0.55));
#5140=CARTESIAN_POINT('',(10.,-0.365,-0.245));
#5141=CARTESIAN_POINT('Origin',(-0.1,-0.82,-0.55));
#5142=CARTESIAN_POINT('',(0.,-0.82,-0.55));
#5143=CARTESIAN_POINT('',(0.,-0.41,-0.55));
#5144=CARTESIAN_POINT('',(10.,-0.82,-0.55));
#5145=CARTESIAN_POINT('',(-0.1,-0.82,-0.55));
#5146=CARTESIAN_POINT('',(10.,-0.41,-0.55));
#5147=CARTESIAN_POINT('Origin',(-0.1,-0.82,-0.3));
#5148=CARTESIAN_POINT('',(0.,-0.82,-0.3));
#5149=CARTESIAN_POINT('',(0.,-0.82,-0.15));
#5150=CARTESIAN_POINT('',(10.,-0.82,-0.3));
#5151=CARTESIAN_POINT('',(-0.1,-0.82,-0.3));
#5152=CARTESIAN_POINT('',(10.,-0.82,-0.15));
#5153=CARTESIAN_POINT('Origin',(-0.1,-1.05,-0.3));
#5154=CARTESIAN_POINT('',(0.,-1.,-0.3));
#5155=CARTESIAN_POINT('',(0.,-0.525,-0.3));
#5156=CARTESIAN_POINT('',(10.,-1.,-0.3));
#5157=CARTESIAN_POINT('',(-0.05,-1.,-0.3));
#5158=CARTESIAN_POINT('',(10.,-0.525,-0.3));
#5159=CARTESIAN_POINT('Origin',(-0.1,0.3,0.82));
#5160=CARTESIAN_POINT('',(0.,0.3,0.82));
#5161=CARTESIAN_POINT('',(0.,0.3,1.));
#5162=CARTESIAN_POINT('',(0.,0.3,0.41));
#5163=CARTESIAN_POINT('',(10.,0.3,0.82));
#5164=CARTESIAN_POINT('',(-0.1,0.3,0.82));
#5165=CARTESIAN_POINT('',(10.,0.3,1.));
#5166=CARTESIAN_POINT('',(10.,0.3,0.41));
#5167=CARTESIAN_POINT('',(-0.05,0.3,1.));
#5168=CARTESIAN_POINT('Origin',(-0.1,0.55,0.82));
#5169=CARTESIAN_POINT('',(0.,0.55,0.82));
#5170=CARTESIAN_POINT('',(0.,0.275,0.82));
#5171=CARTESIAN_POINT('',(10.,0.55,0.82));
#5172=CARTESIAN_POINT('',(-0.1,0.55,0.82));
#5173=CARTESIAN_POINT('',(10.,0.275,0.82));
#5174=CARTESIAN_POINT('Origin',(-0.1,0.55,0.67));
#5175=CARTESIAN_POINT('',(0.,0.55,0.67));
#5176=CARTESIAN_POINT('',(0.,0.55,0.335));
#5177=CARTESIAN_POINT('',(10.,0.55,0.67));
#5178=CARTESIAN_POINT('',(-0.1,0.55,0.67));
#5179=CARTESIAN_POINT('',(10.,0.55,0.335));
#5180=CARTESIAN_POINT('Origin',(-0.1,0.3,0.42));
#5181=CARTESIAN_POINT('',(0.,0.3,0.42));
#5182=CARTESIAN_POINT('',(6.93889390390723E-18,0.12,0.24));
#5183=CARTESIAN_POINT('',(10.,0.3,0.42));
#5184=CARTESIAN_POINT('',(-0.1,0.3,0.42));
#5185=CARTESIAN_POINT('',(10.,0.12,0.24));
#5186=CARTESIAN_POINT('Origin',(-0.1,-0.3,0.42));
#5187=CARTESIAN_POINT('',(0.,-0.3,0.42));
#5188=CARTESIAN_POINT('',(0.,-0.15,0.42));
#5189=CARTESIAN_POINT('',(10.,-0.3,0.42));
#5190=CARTESIAN_POINT('',(-0.1,-0.3,0.42));
#5191=CARTESIAN_POINT('',(10.,-0.15,0.42));
#5192=CARTESIAN_POINT('Origin',(-0.1,-0.55,0.67));
#5193=CARTESIAN_POINT('',(0.,-0.55,0.67));
#5194=CARTESIAN_POINT('',(6.93889390390723E-18,-0.245,0.365));
#5195=CARTESIAN_POINT('',(10.,-0.55,0.67));
#5196=CARTESIAN_POINT('',(-0.1,-0.55,0.67));
#5197=CARTESIAN_POINT('',(10.,-0.245,0.365));
#5198=CARTESIAN_POINT('Origin',(-0.1,-0.55,0.82));
#5199=CARTESIAN_POINT('',(0.,-0.55,0.82));
#5200=CARTESIAN_POINT('',(0.,-0.55,0.41));
#5201=CARTESIAN_POINT('',(10.,-0.55,0.82));
#5202=CARTESIAN_POINT('',(-0.1,-0.55,0.82));
#5203=CARTESIAN_POINT('',(10.,-0.55,0.41));
#5204=CARTESIAN_POINT('Origin',(-0.1,-0.3,0.82));
#5205=CARTESIAN_POINT('',(0.,-0.3,0.82));
#5206=CARTESIAN_POINT('',(0.,-0.15,0.82));
#5207=CARTESIAN_POINT('',(10.,-0.3,0.82));
#5208=CARTESIAN_POINT('',(-0.1,-0.3,0.82));
#5209=CARTESIAN_POINT('',(10.,-0.15,0.82));
#5210=CARTESIAN_POINT('Origin',(-0.1,-0.3,1.05));
#5211=CARTESIAN_POINT('',(0.,-0.3,1.));
#5212=CARTESIAN_POINT('',(0.,-0.3,0.525));
#5213=CARTESIAN_POINT('',(10.,-0.3,1.));
#5214=CARTESIAN_POINT('',(-0.05,-0.3,1.));
#5215=CARTESIAN_POINT('',(10.,-0.3,0.525));
#5216=CARTESIAN_POINT('Origin',(-0.1,0.,0.));
#5217=CARTESIAN_POINT('',(0.,-2.57175827820944E-17,0.21));
#5218=CARTESIAN_POINT('Origin',(0.,0.,0.));
#5219=CARTESIAN_POINT('',(10.,2.57175827820944E-17,0.21));
#5220=CARTESIAN_POINT('',(-0.1,-2.57175827820944E-17,0.21));
#5221=CARTESIAN_POINT('Origin',(10.,0.,0.));
#5222=CARTESIAN_POINT('Origin',(0.,1.,-1.));
#5223=CARTESIAN_POINT('',(0.,1.,1.));
#5224=CARTESIAN_POINT('',(0.,1.,-1.));
#5225=CARTESIAN_POINT('',(10.,1.,1.));
#5226=CARTESIAN_POINT('',(0.,1.,1.));
#5227=CARTESIAN_POINT('',(10.,1.,-1.));
#5228=CARTESIAN_POINT('Origin',(0.,1.,-1.));
#5229=CARTESIAN_POINT('',(10.,1.,-1.));
#5230=CARTESIAN_POINT('',(10.,1.,-1.));
#5231=CARTESIAN_POINT('',(0.,1.,-1.));
#5232=CARTESIAN_POINT('',(0.,1.,-1.));
#5233=CARTESIAN_POINT('',(0.,1.,-1.));
#5234=CARTESIAN_POINT('Origin',(0.,-1.,-1.));
#5235=CARTESIAN_POINT('',(0.,-1.,-1.));
#5236=CARTESIAN_POINT('',(10.,-1.,-1.));
#5237=CARTESIAN_POINT('Origin',(0.,-1.,-1.));
#5238=CARTESIAN_POINT('',(10.,-1.,-1.));
#5239=CARTESIAN_POINT('',(10.,-1.,-1.));
#5240=CARTESIAN_POINT('',(0.,-1.,-1.));
#5241=CARTESIAN_POINT('',(0.,-1.,-1.));
#5242=CARTESIAN_POINT('',(0.,-1.,-1.));
#5243=CARTESIAN_POINT('Origin',(0.,-1.,1.));
#5244=CARTESIAN_POINT('',(0.,-1.,1.));
#5245=CARTESIAN_POINT('',(10.,-1.,1.));
#5246=CARTESIAN_POINT('Origin',(0.,-1.,1.));
#5247=CARTESIAN_POINT('',(10.,-1.,1.));
#5248=CARTESIAN_POINT('',(10.,-1.,1.));
#5249=CARTESIAN_POINT('',(0.,-1.,1.));
#5250=CARTESIAN_POINT('',(0.,-1.,1.));
#5251=CARTESIAN_POINT('',(0.,-1.,1.));
#5252=CARTESIAN_POINT('Origin',(0.,1.,1.));
#5253=CARTESIAN_POINT('',(0.,1.,1.));
#5254=CARTESIAN_POINT('',(10.,1.,1.));
#5255=CARTESIAN_POINT('Origin',(0.,1.,1.));
#5256=CARTESIAN_POINT('',(10.,1.,1.));
#5257=CARTESIAN_POINT('',(0.,1.,1.));
#5258=CARTESIAN_POINT('Origin',(10.,0.,0.));
#5259=CARTESIAN_POINT('Origin',(0.,0.,0.));
#5736=UNCERTAINTY_MEASURE_WITH_UNIT(LENGTH_MEASURE(0.001),#5762,
'DISTANCE_ACCURACY_VALUE',
'Maximum model space distance between geometric entities at asserted c
onnectivities');
#5745=UNCERTAINTY_MEASURE_WITH_UNIT(LENGTH_MEASURE(0.001),#5762,
'DISTANCE_ACCURACY_VALUE',
'Maximum model space distance between geometric entities at asserted c
onnectivities');
#5752=(
GEOMETRIC_REPRESENTATION_CONTEXT(3)
GLOBAL_UNCERTAINTY_ASSIGNED_CONTEXT((#5736))
GLOBAL_UNIT_ASSIGNED_CONTEXT((#5762,#5764,#5765))
REPRESENTATION_CONTEXT('','3D')
);
#5761=(
GEOMETRIC_REPRESENTATION_CONTEXT(3)
GLOBAL_UNCERTAINTY_ASSIGNED_CONTEXT((#5745))
GLOBAL_UNIT_ASSIGNED_CONTEXT((#5762,#5764,#5765))
REPRESENTATION_CONTEXT('','3D')
);
#5762=(
LENGTH_UNIT()
NAMED_UNIT(*)
SI_UNIT(.CENTI.,.METRE.)
);
#5764=(
NAMED_UNIT(*)
PLANE_ANGLE_UNIT()
SI_UNIT($,.RADIAN.)
);
#5765=(
NAMED_UNIT(*)
SI_UNIT($,.STERADIAN.)
SOLID_ANGLE_UNIT()
);
#5772=SHAPE_DEFINITION_REPRESENTATION(#5787,#5821);
#5787=PRODUCT_DEFINITION_SHAPE('',$,#5837);
#5821=SHAPE_REPRESENTATION('',(#3558),#5752);
#5830=PRODUCT_DEFINITION_CONTEXT('part definition',#5877,'design');
#5837=PRODUCT_DEFINITION('Slotted Extrusion - 20 x 20 x 100 mm',
'Slotted Extrusion - 20 x 20 x 100 mm',#5852,#5830);
#5852=PRODUCT_DEFINITION_FORMATION('',$,#5885);
#5877=APPLICATION_CONTEXT(
'Core Data for Automotive Mechanical Design Process');
#5878=PRODUCT_CONTEXT('part definition',#5877,'mechanical');
#5885=PRODUCT('Slotted Extrusion - 20 x 20 x 100 mm',
'Slotted Extrusion - 20 x 20 x 100 mm',
'Slotted Extrusion - 20 x 20 x 100 mm',(#5878));
#5957=COLOUR_RGB('Off White',0.89,0.88,0.83);
#5958=FILL_AREA_STYLE_COLOUR('',#5957);
#5959=FILL_AREA_STYLE('',(#5958));
#5960=SURFACE_STYLE_FILL_AREA(#5959);
#5961=SURFACE_SIDE_STYLE('',(#5960));
#5962=SURFACE_STYLE_USAGE(.BOTH.,#5961);
#5963=PRESENTATION_STYLE_ASSIGNMENT((#5962));
ENDSEC;
END-ISO-10303-21;
